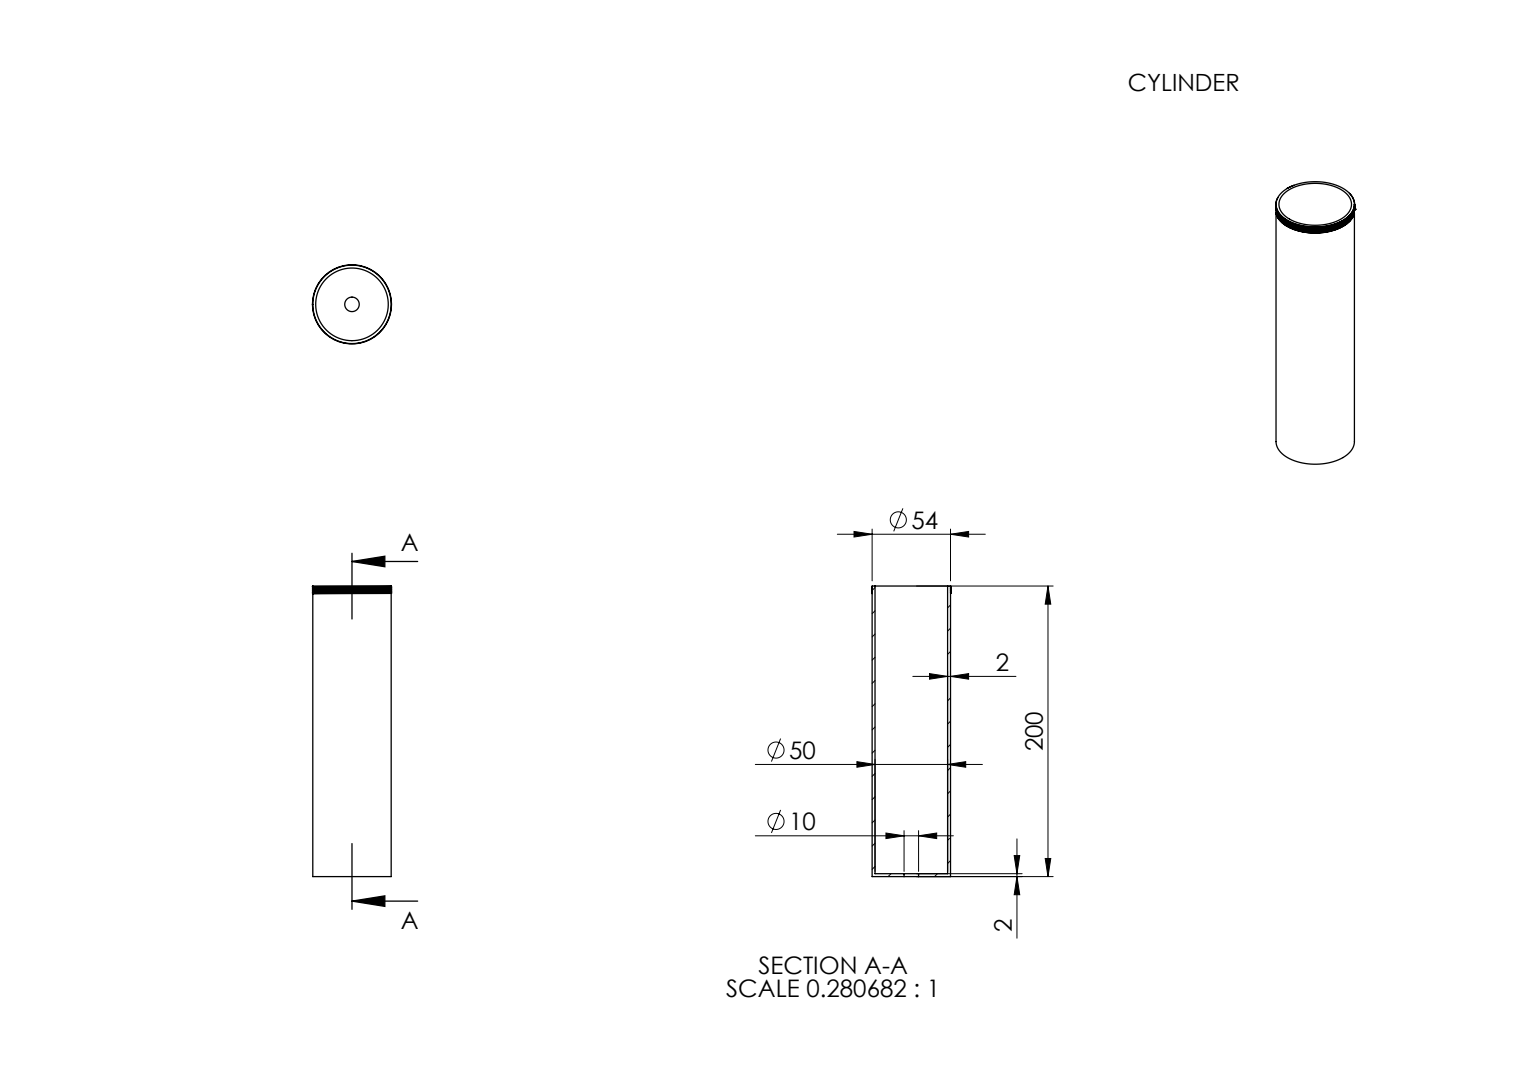
ISO-10303-21;
HEADER;
FILE_DESCRIPTION (('STEP AP214'),
    '1' );
FILE_NAME ('Cylinder.step',
    '2026-10-31T03:36:27',
    ( '' ),
    ( '' ),
    'SwSTEP 2.0',
    'SolidWorks 2026',
    '' );
FILE_SCHEMA (( 'AUTOMOTIVE_DESIGN' ));
ENDSEC;

DATA;
#6=CARTESIAN_POINT ( 'NONE',  ( -3.253724281355068545E-15, 198.6500000012290172, -27.00000000000000355 ) ) ;
#13=CARTESIAN_POINT ( 'NONE',  ( -1.926257025242585782E-15, 198.3968750006145285, -31.45816453501076637 ) ) ;
#14=ORIENTED_EDGE ( 'NONE', *, *, #10865, .F. ) ;
#23=CARTESIAN_POINT ( 'NONE',  ( -13.62178482187500528, 199.2781250006145228, -23.59362340125807123 ) ) ;
#44=CARTESIAN_POINT ( 'NONE',  ( 13.62178482187501416, 195.9593750006145569, 23.59362340125806767 ) ) ;
#51=VECTOR ( 'NONE', #30355, 1000.000000000000000 ) ;
#55=VERTEX_POINT ( 'NONE', #18167 ) ;
#61=CARTESIAN_POINT ( 'NONE',  ( 27.00000000000001066, 196.1375000000000171, 15.58845726811988897 ) ) ;
#84=ORIENTED_EDGE ( 'NONE', *, *, #36303, .T. ) ;
#90=( BOUNDED_CURVE ( )  B_SPLINE_CURVE ( 2, ( #11851, #8830, #29090, #22871, #2761, #17369, #11485, #23054, #34600 ),
 .UNSPECIFIED., .F., .F. ) 
 B_SPLINE_CURVE_WITH_KNOTS ( ( 3, 2, 2, 2, 3 ),
 ( 0.3125000000000000000, 0.3194444444444444198, 0.3333333333333333148, 0.3472222222222222099, 0.3541666666666666852 ),
 .UNSPECIFIED. ) 
 CURVE ( )  GEOMETRIC_REPRESENTATION_ITEM ( )  RATIONAL_B_SPLINE_CURVE ( ( 0.9330127018922194093, 0.9330127018922194093, 1.000000000000000000, 0.8660254037844387076, 1.000000000000000000, 0.8660254037844387076, 1.000000000000000000, 0.9330127018922190762, 0.9330127018922194093 ) ) 
 REPRESENTATION_ITEM ( '' )  );
#93=CARTESIAN_POINT ( 'NONE',  ( 27.24356964375000700, 199.0906250006145228, 15.72908226750537075 ) ) ;
#170=CARTESIAN_POINT ( 'NONE',  ( 5.727106289114498080E-15, 197.0750000012290570, 31.17691453623979214 ) ) ;
#185=CARTESIAN_POINT ( 'NONE',  ( 0.000000000000000000, 2.000000000000000000, 0.000000000000000000 ) ) ;
#199=CARTESIAN_POINT ( 'NONE',  ( 0.000000000000000000, 0.000000000000000000, 0.000000000000000000 ) ) ;
#204=ORIENTED_EDGE ( 'NONE', *, *, #34329, .T. ) ;
#214=CARTESIAN_POINT ( 'NONE',  ( 27.24356964374999635, 199.1656250006145399, -15.72908226750539029 ) ) ;
#226=AXIS2_PLACEMENT_3D ( 'NONE', #11748, #5679, #26519 ) ;
#235=CARTESIAN_POINT ( 'NONE',  ( 13.62178482187501416, 195.0593750006145513, 23.59362340125806767 ) ) ;
#251=CARTESIAN_POINT ( 'NONE',  ( 27.24356964375000345, 198.2843750006145456, -3.336375036156643733E-15 ) ) ;
#256=CARTESIAN_POINT ( 'NONE',  ( -27.00000000000000355, 195.5000000000000000, 0.000000000000000000 ) ) ;
#263=SHAPE_REPRESENTATION_RELATIONSHIP ( 'NONE' , 'NONE' ,  #10836, #22840 ) ;
#296=CARTESIAN_POINT ( 'NONE',  ( 5.727106289114498080E-15, 199.2125000000000057, 31.17691453623979214 ) ) ;
#302=DIRECTION ( 'NONE',  ( -0.000000000000000000, -1.000000000000000000, -0.000000000000000000 ) ) ;
#305=DIRECTION ( 'NONE',  ( 0.000000000000000000, -1.000000000000000000, 0.000000000000000000 ) ) ;
#333=CARTESIAN_POINT ( 'NONE',  ( 26.99999999999999645, 199.8125000000000000, -15.58845726811990495 ) ) ;
#349=ORIENTED_EDGE ( 'NONE', *, *, #34489, .T. ) ;
#357=CARTESIAN_POINT ( 'NONE',  ( 13.49999999999999645, 196.3625000012290513, -23.38268590217984766 ) ) ;
#388=CARTESIAN_POINT ( 'NONE',  ( 27.24356964374999279, 199.2218750006145171, -15.72908226750539207 ) ) ;
#398=CARTESIAN_POINT ( 'NONE',  ( -27.24356964375000345, 198.4531250006145342, 0.000000000000000000 ) ) ;
#420=CARTESIAN_POINT ( 'NONE',  ( 27.24356964375000700, 195.5468750006145342, 15.72908226750537075 ) ) ;
#438=CARTESIAN_POINT ( 'NONE',  ( -27.24356964375000345, 198.0593750006145513, 0.000000000000000000 ) ) ;
#481=CARTESIAN_POINT ( 'NONE',  ( -1.909035429704832693E-15, 199.8875000000000171, -31.17691453623979214 ) ) ;
#539=CARTESIAN_POINT ( 'NONE',  ( 13.50000000000001421, 197.1125000012290513, 23.38268590217984055 ) ) ;
#559=CARTESIAN_POINT ( 'NONE',  ( -27.24356964374999635, 195.8468750006145171, 15.72908226750539384 ) ) ;
#570=CARTESIAN_POINT ( 'NONE',  ( -27.24356964375000345, 198.9218750006145626, -15.72908226750537786 ) ) ;
#580=CARTESIAN_POINT ( 'NONE',  ( -1.926257025242585782E-15, 199.2406250006145285, -31.45816453501075927 ) ) ;
#604=CARTESIAN_POINT ( 'NONE',  ( 27.24356964374999635, 195.6218750006145228, -15.72908226750539029 ) ) ;
#621=CARTESIAN_POINT ( 'NONE',  ( 13.62178482187501416, 197.7593750006145399, 23.59362340125806767 ) ) ;
#665=CARTESIAN_POINT ( 'NONE',  ( -13.50000000000000533, 199.9250000000000114, -23.38268590217984411 ) ) ;
#669=CARTESIAN_POINT ( 'NONE',  ( 0.000000000000000000, 200.0000000000000000, -25.00000000000000000 ) ) ;
#672=CARTESIAN_POINT ( 'NONE',  ( -13.50000000000000533, 198.2375000012290229, -23.38268590217984411 ) ) ;
#725=CARTESIAN_POINT ( 'NONE',  ( 13.49999999999999645, 195.0125000012290570, -23.38268590217984766 ) ) ;
#728=EDGE_CURVE ( 'NONE', #34798, #36105, #17305, .T. ) ;
#748=CARTESIAN_POINT ( 'NONE',  ( 27.24356964375000345, 196.4843750006145626, -3.336375036156643733E-15 ) ) ;
#759=CARTESIAN_POINT ( 'NONE',  ( 0.000000000000000000, 200.0000000000000000, 0.000000000000000000 ) ) ;
#761=CARTESIAN_POINT ( 'NONE',  ( -13.62178482187498396, 196.7843750006145456, 23.59362340125808188 ) ) ;
#774=CARTESIAN_POINT ( 'NONE',  ( 5.778771075727756162E-15, 197.6656250006145399, 31.45816453501075927 ) ) ;
#798=CARTESIAN_POINT ( 'NONE',  ( 13.62178482187501416, 197.7031250006145342, 23.59362340125806767 ) ) ;
#812=CARTESIAN_POINT ( 'NONE',  ( -13.62178482187500528, 197.5343750006145456, -23.59362340125807123 ) ) ;
#813=EDGE_LOOP ( 'NONE', ( #35823, #32630, #11265, #6472 ) ) ;
#817=CARTESIAN_POINT ( 'NONE',  ( -13.49999999999998401, 195.5749999999999886, 23.38268590217985476 ) ) ;
#840=CARTESIAN_POINT ( 'NONE',  ( 27.24356964375000345, 198.6781250006145569, -3.336375036156643733E-15 ) ) ;
#857=CARTESIAN_POINT ( 'NONE',  ( 26.99999999999999645, 199.3625000000000114, -15.58845726811990495 ) ) ;
#872=LINE ( 'NONE', #24196, #29464 ) ;
#896=CARTESIAN_POINT ( 'NONE',  ( 3.306546357697854128E-15, 200.0000000000000000, 27.00000000000000355 ) ) ;
#939=CARTESIAN_POINT ( 'NONE',  ( 5.778771075727756162E-15, 195.0218750006145569, 31.45816453501075927 ) ) ;
#948=CARTESIAN_POINT ( 'NONE',  ( 7.234628195640322446, 198.3325961894323370, 26.99999999999999645 ) ) ;
#950=CARTESIAN_POINT ( 'NONE',  ( -1.926257025242585782E-15, 196.5968750006145456, -31.45816453501076637 ) ) ;
#958=CARTESIAN_POINT ( 'NONE',  ( 3.253724281355069334E-15, 199.5500000012290513, -27.00000000000000000 ) ) ;
#962=CARTESIAN_POINT ( 'NONE',  ( -27.24356964375000345, 196.2031250006145342, 0.000000000000000000 ) ) ;
#985=CARTESIAN_POINT ( 'NONE',  ( 13.62178482187499640, 197.4031250006145228, -23.59362340125807123 ) ) ;
#1023=CARTESIAN_POINT ( 'NONE',  ( 0.000000000000000000, 0.000000000000000000, 0.000000000000000000 ) ) ;
#1027=CARTESIAN_POINT ( 'NONE',  ( 27.24356964374999279, 198.2656250006145058, -15.72908226750539207 ) ) ;
#1039=DIRECTION ( 'NONE',  ( 0.000000000000000000, 0.000000000000000000, -1.000000000000000000 ) ) ;
#1050=CARTESIAN_POINT ( 'NONE',  ( -13.49999999999998401, 198.3875000012290286, 23.38268590217985476 ) ) ;
#1060=EDGE_CURVE ( 'NONE', #37392, #27477, #5776, .T. ) ;
#1101=VERTEX_POINT ( 'NONE', #20197 ) ;
#1124=CARTESIAN_POINT ( 'NONE',  ( -27.00000000000000355, 199.0625000000000000, -15.58845726811989429 ) ) ;
#1128=CARTESIAN_POINT ( 'NONE',  ( -13.62178482187500528, 195.2843750006145456, -23.59362340125807123 ) ) ;
#1135=CARTESIAN_POINT ( 'NONE',  ( 7.234628195640312676, 199.5299038117966859, -27.00000000000000711 ) ) ;
#1136=CARTESIAN_POINT ( 'NONE',  ( 7.234628195640322446, 198.7825961894323257, 26.99999999999999645 ) ) ;
#1138=CARTESIAN_POINT ( 'NONE',  ( -13.62178482187498396, 196.3343750006145285, 23.59362340125808188 ) ) ;
#1139=ORIENTED_EDGE ( 'NONE', *, *, #3630, .F. ) ;
#1150=EDGE_LOOP ( 'NONE', ( #1703, #18410, #14, #35728 ) ) ;
#1151=CARTESIAN_POINT ( 'NONE',  ( -27.24356964375000345, 195.7531250006145456, 0.000000000000000000 ) ) ;
#1174=CARTESIAN_POINT ( 'NONE',  ( -13.62178482187500528, 199.7281250006145399, -23.59362340125807123 ) ) ;
#1177=DIRECTION ( 'NONE',  ( -0.000000000000000000, -1.000000000000000000, -0.000000000000000000 ) ) ;
#1188=ORIENTED_EDGE ( 'NONE', *, *, #28113, .F. ) ;
#1209=CARTESIAN_POINT ( 'NONE',  ( -7.234628195640316228, 197.3200961906614168, -27.00000000000000000 ) ) ;
#1212=CARTESIAN_POINT ( 'NONE',  ( -27.24356964375000345, 197.9656250006145797, -15.72908226750537786 ) ) ;
#1228=CARTESIAN_POINT ( 'NONE',  ( 13.50000000000001421, 198.8000000000000114, 23.38268590217984055 ) ) ;
#1242=ADVANCED_FACE ( 'NONE', ( #35518 ), #20758, .F. ) ;
#1258=CARTESIAN_POINT ( 'NONE',  ( -1.045839947578415010E-13, 196.1750000012290229, 27.00000000000000355 ) ) ;
#1318=VERTEX_POINT ( 'NONE', #35323 ) ;
#1325=CARTESIAN_POINT ( 'NONE',  ( 27.00000000000000355, 199.4375000012290400, -3.306546357697854128E-15 ) ) ;
#1329=CARTESIAN_POINT ( 'NONE',  ( 27.24356964375000700, 195.9968750006145513, 15.72908226750537075 ) ) ;
#1341=CARTESIAN_POINT ( 'NONE',  ( -27.24356964375000345, 196.6531250006145513, 0.000000000000000000 ) ) ;
#1352=FACE_OUTER_BOUND ( 'NONE', #34745, .T. ) ;
#1367=CARTESIAN_POINT ( 'NONE',  ( -27.24356964374999990, 198.8656250006145569, -15.72908226750537786 ) ) ;
#1371=EDGE_CURVE ( 'NONE', #27477, #5428, #18984, .T. ) ;
#1396=CARTESIAN_POINT ( 'NONE',  ( -27.00000000000000355, 198.1625000000000227, -15.58845726811989429 ) ) ;
#1403=CARTESIAN_POINT ( 'NONE',  ( -1.926257025242585782E-15, 198.3406250006145228, -31.45816453501076637 ) ) ;
#1418=CARTESIAN_POINT ( 'NONE',  ( -26.99999999999998934, 196.4375000000000284, 15.58845726811991561 ) ) ;
#1476=ORIENTED_EDGE ( 'NONE', *, *, #2642, .F. ) ;
#1484=CARTESIAN_POINT ( 'NONE',  ( -1.909035429704832693E-15, 195.0500000012290229, -31.17691453623979214 ) ) ;
#1492=CARTESIAN_POINT ( 'NONE',  ( 13.50000000000001421, 196.1000000000000227, 23.38268590217984055 ) ) ;
#1497=DIRECTION ( 'NONE',  ( -0.000000000000000000, -1.000000000000000000, -0.000000000000000000 ) ) ;
#1513=CARTESIAN_POINT ( 'NONE',  ( 27.24356964374999279, 196.5218750006145569, -15.72908226750539207 ) ) ;
#1520=( BOUNDED_CURVE ( )  B_SPLINE_CURVE ( 2, ( #4940, #16154, #15967, #30924, #13483, #25039, #33392, #36780, #7432 ),
 .UNSPECIFIED., .F., .F. ) 
 B_SPLINE_CURVE_WITH_KNOTS ( ( 3, 2, 2, 2, 3 ),
 ( 0.1041666666666666713, 0.1111111111111111049, 0.1250000000000000000, 0.1388888888888888951, 0.1458333333333333426 ),
 .UNSPECIFIED. ) 
 CURVE ( )  GEOMETRIC_REPRESENTATION_ITEM ( )  RATIONAL_B_SPLINE_CURVE ( ( 0.9330127018922194093, 0.9330127018922194093, 1.000000000000000000, 0.8660254037844387076, 1.000000000000000000, 0.8660254037844387076, 1.000000000000000000, 0.9330127018922194093, 0.9330127018922194093 ) ) 
 REPRESENTATION_ITEM ( '' )  );
#1525=CARTESIAN_POINT ( 'NONE',  ( -27.24356964375000345, 197.1031250006145399, 0.000000000000000000 ) ) ;
#1540=DIRECTION ( 'NONE',  ( 0.000000000000000000, -1.000000000000000000, 0.000000000000000000 ) ) ;
#1547=ORIENTED_EDGE ( 'NONE', *, *, #13873, .F. ) ;
#1548=LINE ( 'NONE', #19197, #28798 ) ;
#1552=CARTESIAN_POINT ( 'NONE',  ( -1.926257025242585782E-15, 199.6906250006145456, -31.45816453501075927 ) ) ;
#1565=AXIS2_PLACEMENT_3D ( 'NONE', #36851, #23023, #17153 ) ;
#1580=CARTESIAN_POINT ( 'NONE',  ( 13.50000000000001421, 195.7625000012290570, 23.38268590217984055 ) ) ;
#1593=CARTESIAN_POINT ( 'NONE',  ( -1.926257025242585782E-15, 196.5406250006145399, -31.45816453501076637 ) ) ;
#1595=DIRECTION ( 'NONE',  ( 0.000000000000000000, 0.000000000000000000, -1.000000000000000000 ) ) ;
#1598=CARTESIAN_POINT ( 'NONE',  ( 27.00000000000001421, 196.2500000012290116, 15.58845726811988897 ) ) ;
#1609=CARTESIAN_POINT ( 'NONE',  ( 26.99999999999999645, 198.4625000000000341, -15.58845726811990495 ) ) ;
#1617=CARTESIAN_POINT ( 'NONE',  ( -27.00000000000000355, 196.3625000000000114, -15.58845726811989429 ) ) ;
#1641=DIRECTION ( 'NONE',  ( -0.000000000000000000, -1.000000000000000000, -0.000000000000000000 ) ) ;
#1655=CARTESIAN_POINT ( 'NONE',  ( 6.123233995736766282E-16, 0.000000000000000000, 5.000000000000000000 ) ) ;
#1665=EDGE_LOOP ( 'NONE', ( #22970, #4177, #13653, #15801, #24714, #31155, #33788, #28685 ) ) ;
#1684=CARTESIAN_POINT ( 'NONE',  ( -13.49999999999998401, 195.6875000012290400, 23.38268590217985476 ) ) ;
#1686=DIRECTION ( 'NONE',  ( -0.000000000000000000, -1.000000000000000000, -0.000000000000000000 ) ) ;
#1701=CARTESIAN_POINT ( 'NONE',  ( 5.778771075727756162E-15, 195.9218750006145342, 31.45816453501076637 ) ) ;
#1703=ORIENTED_EDGE ( 'NONE', *, *, #14020, .T. ) ;
#1714=CARTESIAN_POINT ( 'NONE',  ( -27.24356964375001056, 194.8294844423495533, -9.915847621322177119 ) ) ;
#1731=CARTESIAN_POINT ( 'NONE',  ( 13.49999999999999645, 198.0500000000000114, -23.38268590217984766 ) ) ;
#1735=ORIENTED_EDGE ( 'NONE', *, *, #15718, .F. ) ;
#1740=CARTESIAN_POINT ( 'NONE',  ( -13.62178482187500528, 197.0281250006145228, -23.59362340125807123 ) ) ;
#1744=DIRECTION ( 'NONE',  ( 0.000000000000000000, 0.000000000000000000, -1.000000000000000000 ) ) ;
#1761=( BOUNDED_CURVE ( )  B_SPLINE_CURVE ( 2, ( #33202, #15774, #36034, #10078, #28067, #7429, #33389, #27880, #10632 ),
 .UNSPECIFIED., .F., .F. ) 
 B_SPLINE_CURVE_WITH_KNOTS ( ( 3, 2, 2, 2, 3 ),
 ( 0.7708333333333333703, 0.7777777777777777901, 0.7916666666666666297, 0.8055555555555555802, 0.8125000000000000000 ),
 .UNSPECIFIED. ) 
 CURVE ( )  GEOMETRIC_REPRESENTATION_ITEM ( )  RATIONAL_B_SPLINE_CURVE ( ( 0.9330127018922192983, 0.9330127018922198534, 1.000000000000000000, 0.8660254037844387076, 1.000000000000000000, 0.8660254037844387076, 1.000000000000000000, 0.9330127018922194093, 0.9330127018922194093 ) ) 
 REPRESENTATION_ITEM ( '' )  );
#1780=CARTESIAN_POINT ( 'NONE',  ( -13.62178482187498396, 195.3781250006145171, 23.59362340125808188 ) ) ;
#1781=CARTESIAN_POINT ( 'NONE',  ( -27.24356964375000345, 197.1593750006145456, 0.000000000000000000 ) ) ;
#1791=ADVANCED_FACE ( 'NONE', ( #17077 ), #6254, .F. ) ;
#1796=CARTESIAN_POINT ( 'NONE',  ( 13.50000000000001421, 198.3499999999999943, 23.38268590217984055 ) ) ;
#1837=CARTESIAN_POINT ( 'NONE',  ( 27.00000000000000355, 197.6375000012290286, -3.306546357697854128E-15 ) ) ;
#1851=VERTEX_POINT ( 'NONE', #11381 ) ;
#1901=CARTESIAN_POINT ( 'NONE',  ( -13.49999999999998401, 198.3875000012290286, 23.38268590217985476 ) ) ;
#1914=UNCERTAINTY_MEASURE_WITH_UNIT (LENGTH_MEASURE( 1.000000000000000082E-05 ), #7486, 'distance_accuracy_value', 'NONE');
#1915=DIRECTION ( 'NONE',  ( 0.000000000000000000, 1.000000000000000000, 0.000000000000000000 ) ) ;
#1923=CARTESIAN_POINT ( 'NONE',  ( 27.24356964375000700, 195.4906250006145001, 15.72908226750537075 ) ) ;
#1963=CARTESIAN_POINT ( 'NONE',  ( 27.24356964374999635, 197.8718750006145513, -15.72908226750539029 ) ) ;
#1979=CARTESIAN_POINT ( 'NONE',  ( 13.49999999999999645, 197.5999999999999943, -23.38268590217984766 ) ) ;
#2005=EDGE_LOOP ( 'NONE', ( #16646, #26117 ) ) ;
#2032=DIRECTION ( 'NONE',  ( 0.000000000000000000, 0.000000000000000000, -1.000000000000000000 ) ) ;
#2044=CARTESIAN_POINT ( 'NONE',  ( 1.255007937094097924E-14, 199.4375000000000284, -27.00000000000000000 ) ) ;
#2065=CARTESIAN_POINT ( 'NONE',  ( -26.99999999999999645, 197.3375000000000057, 15.58845726811991561 ) ) ;
#2078=CARTESIAN_POINT ( 'NONE',  ( 5.778771075727756162E-15, 195.4718750006145171, 31.45816453501076637 ) ) ;
#2081=CARTESIAN_POINT ( 'NONE',  ( 26.99999999999999645, 196.7750000012290172, -15.58845726811990495 ) ) ;
#2090=EDGE_LOOP ( 'NONE', ( #4509, #18606, #4185, #1735 ) ) ;
#2091=CARTESIAN_POINT ( 'NONE',  ( 26.99999999999999645, 199.0250000012290457, -15.58845726811990495 ) ) ;
#2111=CARTESIAN_POINT ( 'NONE',  ( 13.62178482187501416, 195.0031250006145456, 23.59362340125806767 ) ) ;
#2137=CARTESIAN_POINT ( 'NONE',  ( -1.045839947578415010E-13, 195.7250000012290343, 27.00000000000000355 ) ) ;
#2145=CARTESIAN_POINT ( 'NONE',  ( -1.045839947578415010E-13, 194.8250000012290570, 27.00000000000000355 ) ) ;
#2148=CARTESIAN_POINT ( 'NONE',  ( -1.926257025242585782E-15, 195.6406250006145342, -31.45816453501076637 ) ) ;
#2149=CARTESIAN_POINT ( 'NONE',  ( 13.62178482187499640, 197.4593750006145285, -23.59362340125807123 ) ) ;
#2152=CARTESIAN_POINT ( 'NONE',  ( 1.120210788295102201E-13, 196.4000000012290741, -27.00000000000000711 ) ) ;
#2164=CARTESIAN_POINT ( 'NONE',  ( 26.99999999999999645, 196.2125000000000057, -15.58845726811990495 ) ) ;
#2205=CARTESIAN_POINT ( 'NONE',  ( 7.234628195640295800, 197.5450961906613827, 27.00000000000001066 ) ) ;
#2239=FACE_OUTER_BOUND ( 'NONE', #20647, .T. ) ;
#2257=CARTESIAN_POINT ( 'NONE',  ( 0.000000000000000000, 200.0000000000000000, 0.000000000000000000 ) ) ;
#2265=B_SPLINE_CURVE_WITH_KNOTS ( 'NONE', 3,
 ( #22801, #8950, #17115, #34351 ),
 .UNSPECIFIED., .F., .F.,
 ( 4, 4 ),
 ( 0.000000000000000000, 1.000000000000000000 ),
 .UNSPECIFIED. ) ;
#2270=DIRECTION ( 'NONE',  ( -0.000000000000000000, -1.000000000000000000, -0.000000000000000000 ) ) ;
#2274=CARTESIAN_POINT ( 'NONE',  ( -13.50000000000000533, 199.1375000012290286, -23.38268590217984411 ) ) ;
#2294=ORIENTED_EDGE ( 'NONE', *, *, #16417, .T. ) ;
#2298=CARTESIAN_POINT ( 'NONE',  ( 27.24356964375000700, 195.9406250006145456, 15.72908226750537075 ) ) ;
#2314=EDGE_CURVE ( 'NONE', #21803, #18034, #2265, .T. ) ;
#2327=ORIENTED_EDGE ( 'NONE', *, *, #19803, .F. ) ;
#2337=CARTESIAN_POINT ( 'NONE',  ( 13.50000000000001421, 194.8625000012290513, 23.38268590217984055 ) ) ;
#2340=CARTESIAN_POINT ( 'NONE',  ( -27.24356964375000700, 194.8294844423495817, -9.915847621322177119 ) ) ;
#2341=CARTESIAN_POINT ( 'NONE',  ( 27.24356964375000700, 199.1468750006145285, 15.72908226750537075 ) ) ;
#2355=DIRECTION ( 'NONE',  ( 0.000000000000000000, 0.000000000000000000, -1.000000000000000000 ) ) ;
#2356=CARTESIAN_POINT ( 'NONE',  ( -1.909035429704832693E-15, 196.2875000000000227, -31.17691453623979214 ) ) ;
#2455=DIRECTION ( 'NONE',  ( 0.000000000000000000, 0.000000000000000000, -1.000000000000000000 ) ) ;
#2458=CARTESIAN_POINT ( 'NONE',  ( -20.86978604919638869, 194.8026013911397740, -17.51182792271053046 ) ) ;
#2464=DIRECTION ( 'NONE',  ( -0.000000000000000000, -1.000000000000000000, -0.000000000000000000 ) ) ;
#2482=CARTESIAN_POINT ( 'NONE',  ( 13.62178482187499640, 195.1531250006145513, -23.59362340125807123 ) ) ;
#2489=ORIENTED_EDGE ( 'NONE', *, *, #31608, .T. ) ;
#2526=CARTESIAN_POINT ( 'NONE',  ( -27.24356964374999990, 197.5718750006145399, -15.72908226750537786 ) ) ;
#2529=CARTESIAN_POINT ( 'NONE',  ( 26.99999999999999645, 195.7625000000000171, -15.58845726811990495 ) ) ;
#2537=CARTESIAN_POINT ( 'NONE',  ( 7.234628195640295800, 197.0950961906613941, 27.00000000000001066 ) ) ;
#2543=CARTESIAN_POINT ( 'NONE',  ( -26.99999999999998934, 195.9875000000000114, 15.58845726811991561 ) ) ;
#2577=CARTESIAN_POINT ( 'NONE',  ( 0.000000000000000000, 0.000000000000000000, 0.000000000000000000 ) ) ;
#2631=VERTEX_POINT ( 'NONE', #27747 ) ;
#2639=CARTESIAN_POINT ( 'NONE',  ( -13.50000000000000533, 197.3375000012290457, -23.38268590217984411 ) ) ;
#2642=EDGE_CURVE ( 'NONE', #34685, #32085, #8558, .T. ) ;
#2665=CARTESIAN_POINT ( 'NONE',  ( -20.86978606573367045, 194.8588513912095266, -17.51182790300216752 ) ) ;
#2668=DIRECTION ( 'NONE',  ( 0.000000000000000000, 0.000000000000000000, -1.000000000000000000 ) ) ;
#2672=CARTESIAN_POINT ( 'NONE',  ( 13.62178482187501416, 198.6593750006145456, 23.59362340125806767 ) ) ;
#2686=DIRECTION ( 'NONE',  ( -0.000000000000000000, -1.000000000000000000, -0.000000000000000000 ) ) ;
#2701=CARTESIAN_POINT ( 'NONE',  ( -13.50000000000000533, 198.6875000012290400, -23.38268590217984411 ) ) ;
#2702=CARTESIAN_POINT ( 'NONE',  ( 13.62178482187499640, 196.1093750006145342, -23.59362340125807123 ) ) ;
#2704=CARTESIAN_POINT ( 'NONE',  ( -27.00000000000000355, 198.6125000000000114, -15.58845726811989429 ) ) ;
#2713=CARTESIAN_POINT ( 'NONE',  ( -26.99999999999999645, 195.9875000000000114, 15.58845726811991561 ) ) ;
#2719=VECTOR ( 'NONE', #15417, 1000.000000000000000 ) ;
#2722=CARTESIAN_POINT ( 'NONE',  ( 13.50000000000001421, 196.1000000000000227, 23.38268590217984055 ) ) ;
#2732=EDGE_CURVE ( 'NONE', #10880, #4926, #27922, .T. ) ;
#2761=CARTESIAN_POINT ( 'NONE',  ( -27.00000000000000355, 197.8625000012290513, 0.000000000000000000 ) ) ;
#2775=VERTEX_POINT ( 'NONE', #5174 ) ;
#2781=CARTESIAN_POINT ( 'NONE',  ( 0.000000000000000000, 2.000000000000000000, -5.000000000000000000 ) ) ;
#2804=AXIS2_PLACEMENT_3D ( 'NONE', #21586, #33689, #2032 ) ;
#2808=ORIENTED_EDGE ( 'NONE', *, *, #7091, .T. ) ;
#2826=CARTESIAN_POINT ( 'NONE',  ( 27.00000000000001066, 197.1500000012290172, 15.58845726811988897 ) ) ;
#2866=CARTESIAN_POINT ( 'NONE',  ( -27.24356964374999635, 198.4906250006145569, 15.72908226750539384 ) ) ;
#2886=CARTESIAN_POINT ( 'NONE',  ( 13.50000000000001421, 195.2000000000000171, 23.38268590217984055 ) ) ;
#2888=CARTESIAN_POINT ( 'NONE',  ( 27.24356964375000700, 196.4468750006145115, 15.72908226750537075 ) ) ;
#2908=CARTESIAN_POINT ( 'NONE',  ( -27.00000000000000355, 195.5000000000000000, 0.000000000000000000 ) ) ;
#2916=EDGE_CURVE ( 'NONE', #24650, #4030, #22848, .T. ) ;
#2957=CARTESIAN_POINT ( 'NONE',  ( -13.50000000000000533, 196.4375000012290400, -23.38268590217984411 ) ) ;
#2974=( BOUNDED_CURVE ( )  B_SPLINE_CURVE ( 2, ( #13003, #16223, #10152, #12806, #15662, #10338, #36478, #25112, #10519 ),
 .UNSPECIFIED., .F., .F. ) 
 B_SPLINE_CURVE_WITH_KNOTS ( ( 3, 2, 2, 2, 3 ),
 ( 0.06250000000000000000, 0.06944444444444444753, 0.08333333333333332871, 0.09722222222222222376, 0.1041666666666666713 ),
 .UNSPECIFIED. ) 
 CURVE ( )  GEOMETRIC_REPRESENTATION_ITEM ( )  RATIONAL_B_SPLINE_CURVE ( ( 0.9330127018922194093, 0.9330127018922194093, 1.000000000000000000, 0.8660254037844387076, 1.000000000000000000, 0.8660254037844387076, 1.000000000000000000, 0.9330127018922192983, 0.9330127018922194093 ) ) 
 REPRESENTATION_ITEM ( '' )  );
#3015=CARTESIAN_POINT ( 'NONE',  ( 27.00000000000001066, 197.6000000012290627, 15.58845726811988897 ) ) ;
#3039=CARTESIAN_POINT ( 'NONE',  ( -27.24356964375000345, 194.8531250006145115, 0.000000000000000000 ) ) ;
#3056=CARTESIAN_POINT ( 'NONE',  ( 13.62178482187499640, 198.3031250006145285, -23.59362340125807123 ) ) ;
#3077=CARTESIAN_POINT ( 'NONE',  ( 13.49999999999999645, 195.3500000000000227, -23.38268590217984766 ) ) ;
#3078=CARTESIAN_POINT ( 'NONE',  ( -27.24356964375000345, 195.3593750006145342, 0.000000000000000000 ) ) ;
#3089=CARTESIAN_POINT ( 'NONE',  ( 13.50000000000001421, 197.1125000012290513, 23.38268590217984055 ) ) ;
#3096=CARTESIAN_POINT ( 'NONE',  ( -13.62178482187498396, 198.1343750006145399, 23.59362340125808188 ) ) ;
#3097=ORIENTED_EDGE ( 'NONE', *, *, #28113, .T. ) ;
#3125=CARTESIAN_POINT ( 'NONE',  ( -27.24356964375000345, 198.8656250006145285, -15.72908226750537786 ) ) ;
#3136=VERTEX_POINT ( 'NONE', #22541 ) ;
#3144=CARTESIAN_POINT ( 'NONE',  ( -7.234628195640263826, 196.4200961906613543, -27.00000000000003553 ) ) ;
#3199=CARTESIAN_POINT ( 'NONE',  ( -27.00000000000000355, 196.0625000012290400, 0.000000000000000000 ) ) ;
#3206=MECHANICAL_DESIGN_GEOMETRIC_PRESENTATION_REPRESENTATION('',(#5694),#13523);
#3211=EDGE_CURVE ( 'NONE', #24650, #1318, #22173, .T. ) ;
#3221=CARTESIAN_POINT ( 'NONE',  ( 13.62178482187501416, 195.0593750006145513, 23.59362340125806767 ) ) ;
#3233=CARTESIAN_POINT ( 'NONE',  ( -1.926257025242585782E-15, 199.2968750006145342, -31.45816453501076637 ) ) ;
#3243=ORIENTED_EDGE ( 'NONE', *, *, #2916, .F. ) ;
#3245=CARTESIAN_POINT ( 'NONE',  ( -27.24356964374999990, 199.7656250006145342, -15.72908226750537786 ) ) ;
#3257=( GEOMETRIC_REPRESENTATION_CONTEXT ( 3 ) GLOBAL_UNCERTAINTY_ASSIGNED_CONTEXT ( ( #1914 ) ) GLOBAL_UNIT_ASSIGNED_CONTEXT ( ( #7486, #36656, #30615 ) ) REPRESENTATION_CONTEXT ( 'NONE', 'WORKASPACE' ) );
#3264=ORIENTED_EDGE ( 'NONE', *, *, #2916, .T. ) ;
#3268=CARTESIAN_POINT ( 'NONE',  ( 27.24356964375000345, 195.5843750006145285, -3.336375036156643733E-15 ) ) ;
#3284=CARTESIAN_POINT ( 'NONE',  ( 5.778771075727756162E-15, 198.1718750006145342, 31.45816453501075927 ) ) ;
#3311=CARTESIAN_POINT ( 'NONE',  ( -13.62178482187500528, 198.8281250006145342, -23.59362340125807123 ) ) ;
#3316=DIRECTION ( 'NONE',  ( -0.000000000000000000, -1.000000000000000000, -0.000000000000000000 ) ) ;
#3329=CARTESIAN_POINT ( 'NONE',  ( 5.727106289114498080E-15, 199.6625000000000227, 31.17691453623979214 ) ) ;
#3335=CARTESIAN_POINT ( 'NONE',  ( 1.069080835302379631E-14, 198.4250000012290229, 27.00000000000000000 ) ) ;
#3376=CARTESIAN_POINT ( 'NONE',  ( 13.50000000000001421, 196.5500000000000114, 23.38268590217984055 ) ) ;
#3386=ADVANCED_FACE ( 'NONE', ( #28394 ), #5091, .T. ) ;
#3392=CARTESIAN_POINT ( 'NONE',  ( 26.99999999999999645, 195.4250000012290229, -15.58845726811990495 ) ) ;
#3410=CARTESIAN_POINT ( 'NONE',  ( 27.24356964375000700, 196.4468750006145115, 15.72908226750537075 ) ) ;
#3422=CARTESIAN_POINT ( 'NONE',  ( -27.24356964374999279, 198.9968750006145513, 15.72908226750539384 ) ) ;
#3432=CARTESIAN_POINT ( 'NONE',  ( -27.24356964375000345, 198.0031250006145456, 0.000000000000000000 ) ) ;
#3449=ORIENTED_EDGE ( 'NONE', *, *, #26598, .T. ) ;
#3454=CARTESIAN_POINT ( 'NONE',  ( -7.234628195640316228, 198.6700961906613543, -27.00000000000000000 ) ) ;
#3456=CARTESIAN_POINT ( 'NONE',  ( 27.24356964375000700, 195.0968750006145456, 15.72908226750537075 ) ) ;
#3474=CARTESIAN_POINT ( 'NONE',  ( -27.24356964374999635, 197.6468750006145285, 15.72908226750539384 ) ) ;
#3476=ORIENTED_EDGE ( 'NONE', *, *, #22471, .T. ) ;
#3495=LINE ( 'NONE', #20761, #21688 ) ;
#3500=CARTESIAN_POINT ( 'NONE',  ( -27.24356964375000345, 199.3531250006145399, 0.000000000000000000 ) ) ;
#3510=ORIENTED_EDGE ( 'NONE', *, *, #36113, .F. ) ;
#3575=ORIENTED_EDGE ( 'NONE', *, *, #31144, .F. ) ;
#3602=CARTESIAN_POINT ( 'NONE',  ( 27.24356964375000345, 195.1343750006145399, -3.336375036156643733E-15 ) ) ;
#3612=CYLINDRICAL_SURFACE ( 'NONE', #31490, 27.00000000000000355 ) ;
#3614=CARTESIAN_POINT ( 'NONE',  ( -27.24356964375000345, 197.5718750006145115, -15.72908226750537786 ) ) ;
#3624=CARTESIAN_POINT ( 'NONE',  ( -13.62178482187500528, 197.9281250006145569, -23.59362340125807123 ) ) ;
#3630=EDGE_CURVE ( 'NONE', #34798, #17216, #32174, .T. ) ;
#3632=CARTESIAN_POINT ( 'NONE',  ( 13.50000000000001421, 197.0000000000000000, 23.38268590217984055 ) ) ;
#3648=CARTESIAN_POINT ( 'NONE',  ( -27.24356964375000345, 198.0031250006145456, 0.000000000000000000 ) ) ;
#3653=DIRECTION ( 'NONE',  ( -0.000000000000000000, -1.000000000000000000, -0.000000000000000000 ) ) ;
#3661=CARTESIAN_POINT ( 'NONE',  ( -1.926257025242585782E-15, 197.0468750006145626, -31.45816453501075927 ) ) ;
#3691=LINE ( 'NONE', #12410, #22908 ) ;
#3782=CARTESIAN_POINT ( 'NONE',  ( 27.24356964375000700, 196.8968750006145285, 15.72908226750537075 ) ) ;
#3784=ORIENTED_EDGE ( 'NONE', *, *, #36113, .T. ) ;
#3793=CARTESIAN_POINT ( 'NONE',  ( -13.62178482187500528, 197.0843750006145285, -23.59362340125807123 ) ) ;
#3794=ORIENTED_EDGE ( 'NONE', *, *, #27314, .F. ) ;
#3806=CARTESIAN_POINT ( 'NONE',  ( -1.926257025242585782E-15, 196.9906250006145569, -31.45816453501075927 ) ) ;
#3833=CARTESIAN_POINT ( 'NONE',  ( -13.62178482187500528, 197.4781250006145399, -23.59362340125807123 ) ) ;
#3834=CARTESIAN_POINT ( 'NONE',  ( 27.00000000000000355, 198.0875000012290457, -3.306546357697854128E-15 ) ) ;
#3863=AXIS2_PLACEMENT_3D ( 'NONE', #4306, #27809, #31209 ) ;
#3875=CARTESIAN_POINT ( 'NONE',  ( 27.24356964375000700, 197.2906250006145399, 15.72908226750537075 ) ) ;
#3887=CARTESIAN_POINT ( 'NONE',  ( 0.000000000000000000, 200.0000000000000000, 0.000000000000000000 ) ) ;
#3894=CARTESIAN_POINT ( 'NONE',  ( 13.50000000000001421, 199.2500000000000000, 23.38268590217984055 ) ) ;
#3897=ORIENTED_EDGE ( 'NONE', *, *, #19583, .F. ) ;
#3900=FACE_OUTER_BOUND ( 'NONE', #18753, .T. ) ;
#3941=ADVANCED_FACE ( 'NONE', ( #18546 ), #26670, .F. ) ;
#3953=CARTESIAN_POINT ( 'NONE',  ( -27.00000000000000355, 195.1625000012290343, 0.000000000000000000 ) ) ;
#3970=CARTESIAN_POINT ( 'NONE',  ( 26.99999999999999645, 199.0250000012290172, -15.58845726811990495 ) ) ;
#3973=CARTESIAN_POINT ( 'NONE',  ( -27.24356964374999635, 196.7468750006145797, 15.72908226750539384 ) ) ;
#3982=CARTESIAN_POINT ( 'NONE',  ( 27.00000000000000355, 198.4250000000000114, -3.306546357697854128E-15 ) ) ;
#3984=CARTESIAN_POINT ( 'NONE',  ( -13.62178482187498396, 198.1343750006145399, 23.59362340125808188 ) ) ;
#3993=ORIENTED_EDGE ( 'NONE', *, *, #36975, .T. ) ;
#3996=CARTESIAN_POINT ( 'NONE',  ( 27.24356964374999635, 196.0156250006145626, -15.72908226750539029 ) ) ;
#4023=CARTESIAN_POINT ( 'NONE',  ( -13.62178482187498396, 198.9781250006145399, 23.59362340125808188 ) ) ;
#4024=CYLINDRICAL_SURFACE ( 'NONE', #12318, 27.00000000000000355 ) ;
#4030=VERTEX_POINT ( 'NONE', #24216 ) ;
#4056=CARTESIAN_POINT ( 'NONE',  ( -7.234628195640289583, 198.1075961894323143, -27.00000000000001421 ) ) ;
#4064=CARTESIAN_POINT ( 'NONE',  ( -27.24356964375000345, 198.0031250006145456, 0.000000000000000000 ) ) ;
#4066=LINE ( 'NONE', #10130, #20503 ) ;
#4090=CARTESIAN_POINT ( 'NONE',  ( -7.234628195640302017, 198.4049038117967143, 27.00000000000000711 ) ) ;
#4118=DIRECTION ( 'NONE',  ( 0.000000000000000000, 0.000000000000000000, -1.000000000000000000 ) ) ;
#4145=CARTESIAN_POINT ( 'NONE',  ( 5.727106289114498080E-15, 195.2750000012290172, 31.17691453623979214 ) ) ;
#4176=CARTESIAN_POINT ( 'NONE',  ( 27.24356964374999279, 196.0718750006145399, -15.72908226750539207 ) ) ;
#4177=ORIENTED_EDGE ( 'NONE', *, *, #27306, .T. ) ;
#4183=( BOUNDED_CURVE ( )  B_SPLINE_CURVE ( 2, ( #2152, #5183, #10876, #27568, #11062, #1598, #34184, #22265, #33439 ),
 .UNSPECIFIED., .F., .F. ) 
 B_SPLINE_CURVE_WITH_KNOTS ( ( 3, 2, 2, 2, 3 ),
 ( 0.6041666666666667407, 0.6111111111111111605, 0.6250000000000000000, 0.6388888888888888395, 0.6458333333333333703 ),
 .UNSPECIFIED. ) 
 CURVE ( )  GEOMETRIC_REPRESENTATION_ITEM ( )  RATIONAL_B_SPLINE_CURVE ( ( 0.9330127018922192983, 0.9330127018922198534, 1.000000000000000000, 0.8660254037844387076, 1.000000000000000000, 0.8660254037844387076, 1.000000000000000000, 0.9330127018922187432, 0.9330127018922192983 ) ) 
 REPRESENTATION_ITEM ( '' )  );
#4185=ORIENTED_EDGE ( 'NONE', *, *, #35475, .F. ) ;
#4188=CARTESIAN_POINT ( 'NONE',  ( 27.24356964375000345, 195.9781250006145399, -3.336375036156643733E-15 ) ) ;
#4210=CARTESIAN_POINT ( 'NONE',  ( 27.24356964374999635, 198.7156250006145513, -15.72908226750539029 ) ) ;
#4211=CARTESIAN_POINT ( 'NONE',  ( -27.00000000000000355, 200.0000000000000000, 0.000000000000000000 ) ) ;
#4249=CARTESIAN_POINT ( 'NONE',  ( -27.24356964375000345, 197.1031250006145399, 0.000000000000000000 ) ) ;
#4253=CARTESIAN_POINT ( 'NONE',  ( -1.045839947578415010E-13, 195.1625000000000512, 27.00000000000000355 ) ) ;
#4265=CARTESIAN_POINT ( 'NONE',  ( 27.00000000000000355, 197.5250000000000057, -3.306546357697854128E-15 ) ) ;
#4288=DIRECTION ( 'NONE',  ( 0.000000000000000000, -1.000000000000000000, 0.000000000000000000 ) ) ;
#4306=CARTESIAN_POINT ( 'NONE',  ( 0.000000000000000000, 200.0000000000000000, 0.000000000000000000 ) ) ;
#4320=AXIS2_PLACEMENT_3D ( 'NONE', #185, #22254, #37331 ) ;
#4328=CARTESIAN_POINT ( 'NONE',  ( 27.00000000000001066, 194.9000000012290457, 15.58845726811988897 ) ) ;
#4349=EDGE_LOOP ( 'NONE', ( #10680, #4641, #36463, #13800 ) ) ;
#4358=CARTESIAN_POINT ( 'NONE',  ( 27.24356964375000700, 197.3468750006145740, 15.72908226750537075 ) ) ;
#4371=ORIENTED_EDGE ( 'NONE', *, *, #15199, .F. ) ;
#4372=CARTESIAN_POINT ( 'NONE',  ( -13.62178482187498396, 197.1781250006145569, 23.59362340125808188 ) ) ;
#4383=VERTEX_POINT ( 'NONE', #37250 ) ;
#4395=CARTESIAN_POINT ( 'NONE',  ( 5.778771075727756162E-15, 197.6656250006145399, 31.45816453501075927 ) ) ;
#4416=( BOUNDED_CURVE ( )  B_SPLINE_CURVE ( 2, ( #6515, #14670, #817, #26220, #256, #11821, #23390, #20555, #37156 ),
 .UNSPECIFIED., .F., .F. ) 
 B_SPLINE_CURVE_WITH_KNOTS ( ( 3, 2, 2, 2, 3 ),
 ( 0.8125000000000000000, 0.8194444444444444198, 0.8333333333333333703, 0.8472222222222222099, 0.8541666666666667407 ),
 .UNSPECIFIED. ) 
 CURVE ( )  GEOMETRIC_REPRESENTATION_ITEM ( )  RATIONAL_B_SPLINE_CURVE ( ( 0.9330127018922194093, 0.9330127018922194093, 1.000000000000000000, 0.8660254037844387076, 1.000000000000000000, 0.8660254037844387076, 1.000000000000000000, 0.9330127018922187432, 0.9330127018922192983 ) ) 
 REPRESENTATION_ITEM ( '' )  );
#4431=DIRECTION ( 'NONE',  ( 0.000000000000000000, 1.000000000000000000, 0.000000000000000000 ) ) ;
#4435=CARTESIAN_POINT ( 'NONE',  ( -27.24356964374999279, 196.6906250006145456, 15.72908226750539384 ) ) ;
#4451=CARTESIAN_POINT ( 'NONE',  ( -26.99999999999998934, 198.6875000000000284, 15.58845726811991561 ) ) ;
#4452=ORIENTED_EDGE ( 'NONE', *, *, #8939, .F. ) ;
#4454=ORIENTED_EDGE ( 'NONE', *, *, #35475, .T. ) ;
#4465=AXIS2_PLACEMENT_3D ( 'NONE', #37028, #37216, #2355 ) ;
#4483=CYLINDRICAL_SURFACE ( 'NONE', #15052, 25.00000000000000000 ) ;
#4509=ORIENTED_EDGE ( 'NONE', *, *, #18682, .T. ) ;
#4532=LINE ( 'NONE', #16293, #34504 ) ;
#4538=ORIENTED_EDGE ( 'NONE', *, *, #36547, .F. ) ;
#4560=CARTESIAN_POINT ( 'NONE',  ( 13.62178482187499640, 196.0531250006145285, -23.59362340125807123 ) ) ;
#4571=ORIENTED_EDGE ( 'NONE', *, *, #13873, .T. ) ;
#4573=CARTESIAN_POINT ( 'NONE',  ( 0.000000000000000000, 0.000000000000000000, 0.000000000000000000 ) ) ;
#4586=CARTESIAN_POINT ( 'NONE',  ( -27.24356964375000345, 197.1031250006145399, 0.000000000000000000 ) ) ;
#4608=CARTESIAN_POINT ( 'NONE',  ( 3.306546357697854128E-15, 200.0000000000000000, 27.00000000000000355 ) ) ;
#4620=ORIENTED_EDGE ( 'NONE', *, *, #20907, .T. ) ;
#4622=CARTESIAN_POINT ( 'NONE',  ( 5.778771075727756162E-15, 198.1156250006145285, 31.45816453501076637 ) ) ;
#4623=CARTESIAN_POINT ( 'NONE',  ( -27.24356964375000345, 199.4093750006145456, 0.000000000000000000 ) ) ;
#4636=CARTESIAN_POINT ( 'NONE',  ( 6.123233995736766282E-16, 2.000000000000000000, 5.000000000000000000 ) ) ;
#4637=CARTESIAN_POINT ( 'NONE',  ( -13.49999999999998401, 197.3750000000000284, 23.38268590217985476 ) ) ;
#4641=ORIENTED_EDGE ( 'NONE', *, *, #36536, .T. ) ;
#4651=DIRECTION ( 'NONE',  ( 0.000000000000000000, 0.000000000000000000, 1.000000000000000000 ) ) ;
#4715=CARTESIAN_POINT ( 'NONE',  ( -7.234628195640263826, 195.5200961906613770, -27.00000000000003553 ) ) ;
#4734=CARTESIAN_POINT ( 'NONE',  ( -27.24356964374999279, 194.9468750006145683, 15.72908226750539384 ) ) ;
#4748=CARTESIAN_POINT ( 'NONE',  ( 27.24356964375000345, 195.0781250006145342, -3.336375036156643733E-15 ) ) ;
#4759=DIRECTION ( 'NONE',  ( -0.000000000000000000, -1.000000000000000000, -0.000000000000000000 ) ) ;
#4771=CARTESIAN_POINT ( 'NONE',  ( 27.24356964374999635, 195.5656250006145171, -15.72908226750539029 ) ) ;
#4786=UNCERTAINTY_MEASURE_WITH_UNIT (LENGTH_MEASURE( 1.000000000000000082E-05 ), #19083, 'distance_accuracy_value', 'NONE');
#4808=CARTESIAN_POINT ( 'NONE',  ( 5.778771075727756162E-15, 198.1718750006145342, 31.45816453501075927 ) ) ;
#4811=CARTESIAN_POINT ( 'NONE',  ( -13.49999999999998401, 195.1250000000000284, 23.38268590217985476 ) ) ;
#4822=CARTESIAN_POINT ( 'NONE',  ( -13.50000000000000533, 196.7750000000000057, -23.38268590217984411 ) ) ;
#4914=LINE ( 'NONE', #5104, #2719 ) ;
#4926=VERTEX_POINT ( 'NONE', #24357 ) ;
#4927=CARTESIAN_POINT ( 'NONE',  ( 27.24356964375000700, 195.0406250006145399, 15.72908226750537075 ) ) ;
#4940=CARTESIAN_POINT ( 'NONE',  ( 1.255007937094097924E-14, 199.4375000000000284, -27.00000000000000000 ) ) ;
#4945=CARTESIAN_POINT ( 'NONE',  ( 0.000000000000000000, 200.0000000000000000, 0.000000000000000000 ) ) ;
#4947=VECTOR ( 'NONE', #1686, 1000.000000000000000 ) ;
#4949=CARTESIAN_POINT ( 'NONE',  ( -27.24356964375000345, 196.2031250006145342, 0.000000000000000000 ) ) ;
#4957=ORIENTED_EDGE ( 'NONE', *, *, #728, .F. ) ;
#4978=CARTESIAN_POINT ( 'NONE',  ( 13.49999999999999645, 195.9125000012290343, -23.38268590217984766 ) ) ;
#4989=CARTESIAN_POINT ( 'NONE',  ( 5.778771075727756162E-15, 195.4156250006145399, 31.45816453501076637 ) ) ;
#4991=CARTESIAN_POINT ( 'NONE',  ( 5.778771075727756162E-15, 199.0718750006145399, 31.45816453501075927 ) ) ;
#5009=CARTESIAN_POINT ( 'NONE',  ( -27.00000000000000355, 198.1625000000000227, -15.58845726811989429 ) ) ;
#5013=VERTEX_POINT ( 'NONE', #19056 ) ;
#5050=CARTESIAN_POINT ( 'NONE',  ( -4.694659320240884604E-14, 197.5250000012290172, 27.00000000000000000 ) ) ;
#5089=CARTESIAN_POINT ( 'NONE',  ( -27.00000000000000355, 195.6125000012290513, 0.000000000000000000 ) ) ;
#5091=CYLINDRICAL_SURFACE ( 'NONE', #14055, 27.00000000000000355 ) ;
#5104=CARTESIAN_POINT ( 'NONE',  ( 3.306546357697854128E-15, 200.0000000000000000, 27.00000000000000355 ) ) ;
#5106=CARTESIAN_POINT ( 'NONE',  ( -27.24356964375000345, 195.7718750006145569, -15.72908226750537786 ) ) ;
#5117=CARTESIAN_POINT ( 'NONE',  ( -13.62178482187498396, 194.9281250006145569, 23.59362340125808188 ) ) ;
#5138=CARTESIAN_POINT ( 'NONE',  ( -27.24356964374999635, 196.2406250006145285, 15.72908226750539384 ) ) ;
#5153=CARTESIAN_POINT ( 'NONE',  ( -13.50000000000000533, 199.9250000000000114, -23.38268590217984411 ) ) ;
#5165=CARTESIAN_POINT ( 'NONE',  ( 0.000000000000000000, 200.0000000000000000, 0.000000000000000000 ) ) ;
#5174=CARTESIAN_POINT ( 'NONE',  ( 0.000000000000000000, 0.000000000000000000, -27.00000000000000355 ) ) ;
#5175=ORIENTED_EDGE ( 'NONE', *, *, #15166, .T. ) ;
#5177=CIRCLE ( 'NONE', #17289, 5.000000000000000000 ) ;
#5178=CARTESIAN_POINT ( 'NONE',  ( -27.24356964374999279, 194.8906250006145342, 15.72908226750539384 ) ) ;
#5179=CARTESIAN_POINT ( 'NONE',  ( -27.24356964374999990, 198.9218750006145626, -15.72908226750537786 ) ) ;
#5182=ADVANCED_FACE ( 'NONE', ( #36646 ), #27566, .T. ) ;
#5183=CARTESIAN_POINT ( 'NONE',  ( 7.234628195640363302, 196.3799038117967086, -26.99999999999996803 ) ) ;
#5197=CARTESIAN_POINT ( 'NONE',  ( -27.00000000000000355, 195.0500000000000114, 0.000000000000000000 ) ) ;
#5222=ORIENTED_EDGE ( 'NONE', *, *, #15718, .T. ) ;
#5230=AXIS2_PLACEMENT_3D ( 'NONE', #5165, #5353, #37001 ) ;
#5238=CARTESIAN_POINT ( 'NONE',  ( 26.99999999999999645, 197.6750000012290229, -15.58845726811990495 ) ) ;
#5255=CARTESIAN_POINT ( 'NONE',  ( 0.000000000000000000, 200.0000000000000000, 0.000000000000000000 ) ) ;
#5276=CARTESIAN_POINT ( 'NONE',  ( -13.62178482187500528, 199.2781250006145228, -23.59362340125807123 ) ) ;
#5298=EDGE_CURVE ( 'NONE', #29410, #26583, #5658, .T. ) ;
#5303=CARTESIAN_POINT ( 'NONE',  ( 13.49999999999999645, 198.6125000012290513, -23.38268590217984766 ) ) ;
#5327=CARTESIAN_POINT ( 'NONE',  ( -13.62178482187498396, 195.3781250006145171, 23.59362340125808188 ) ) ;
#5353=DIRECTION ( 'NONE',  ( -0.000000000000000000, -1.000000000000000000, -0.000000000000000000 ) ) ;
#5362=CARTESIAN_POINT ( 'NONE',  ( 13.62178482187501416, 195.9031250006145513, 23.59362340125806767 ) ) ;
#5363=CARTESIAN_POINT ( 'NONE',  ( 27.24356964374999635, 199.2218750006145456, -15.72908226750539029 ) ) ;
#5365=PLANE ( 'NONE',  #35980 ) ;
#5377=CARTESIAN_POINT ( 'NONE',  ( 13.49999999999999645, 195.8000000000000114, -23.38268590217984766 ) ) ;
#5428=VERTEX_POINT ( 'NONE', #5733 ) ;
#5446=ORIENTED_EDGE ( 'NONE', *, *, #20976, .T. ) ;
#5449=CYLINDRICAL_SURFACE ( 'NONE', #30803, 27.00000000000000355 ) ;
#5476=CARTESIAN_POINT ( 'NONE',  ( -20.68320086892770604, 194.6619763917542798, -17.35526438333879540 ) ) ;
#5480=CARTESIAN_POINT ( 'NONE',  ( 27.00000000000001066, 198.0500000012290513, 15.58845726811988897 ) ) ;
#5499=CARTESIAN_POINT ( 'NONE',  ( 1.255007937094097924E-14, 199.4375000000000284, -27.00000000000000355 ) ) ;
#5529=VERTEX_POINT ( 'NONE', #8037 ) ;
#5530=CARTESIAN_POINT ( 'NONE',  ( -7.234628195640263826, 196.7575961894323484, -27.00000000000003553 ) ) ;
#5542=CARTESIAN_POINT ( 'NONE',  ( -27.24356964375000345, 194.8531250006145115, 0.000000000000000000 ) ) ;
#5543=CARTESIAN_POINT ( 'NONE',  ( -27.24356964374999990, 199.7656250006145342, -15.72908226750537786 ) ) ;
#5546=EDGE_CURVE ( 'NONE', #33961, #26752, #22404, .T. ) ;
#5562=CARTESIAN_POINT ( 'NONE',  ( -1.909035429704832693E-15, 195.3874999999999886, -31.17691453623979214 ) ) ;
#5568=FACE_OUTER_BOUND ( 'NONE', #9147, .T. ) ;
#5600=VERTEX_POINT ( 'NONE', #21295 ) ;
#5626=( BOUNDED_CURVE ( )  B_SPLINE_CURVE ( 2, ( #25808, #16551, #5153, #33971, #19221 ),
 .UNSPECIFIED., .F., .F. ) 
 B_SPLINE_CURVE_WITH_KNOTS ( ( 3, 2, 3 ),
 ( 0.000000000000000000, 0.01388888888888888985, 0.02083333333333333565 ),
 .UNSPECIFIED. ) 
 CURVE ( )  GEOMETRIC_REPRESENTATION_ITEM ( )  RATIONAL_B_SPLINE_CURVE ( ( 1.000000000000000000, 0.8660254037844387076, 1.000000000000000000, 0.9330127018922192983, 0.9330127018922194093 ) ) 
 REPRESENTATION_ITEM ( '' )  );
#5658=CIRCLE ( 'NONE', #15356, 25.00000000000000000 ) ;
#5668=CARTESIAN_POINT ( 'NONE',  ( -26.99999999999998934, 197.0000000012290400, 15.58845726811991561 ) ) ;
#5679=DIRECTION ( 'NONE',  ( 0.000000000000000000, -1.000000000000000000, 0.000000000000000000 ) ) ;
#5694=STYLED_ITEM ( 'NONE', ( #22290 ), #22840 ) ;
#5699=CARTESIAN_POINT ( 'NONE',  ( -27.24356964375000345, 198.9593750006145285, 0.000000000000000000 ) ) ;
#5707=EDGE_CURVE ( 'NONE', #10453, #29410, #9344, .T. ) ;
#5710=CARTESIAN_POINT ( 'NONE',  ( 13.62178482187501416, 199.5031250006145456, 23.59362340125806767 ) ) ;
#5715=ADVANCED_FACE ( 'NONE', ( #29993 ), #4024, .T. ) ;
#5727=( BOUNDED_CURVE ( )  B_SPLINE_CURVE ( 2, ( #15743, #1135, #10045, #21255, #1325, #32604, #21622, #18600, #26723 ),
 .UNSPECIFIED., .F., .F. ) 
 B_SPLINE_CURVE_WITH_KNOTS ( ( 3, 2, 2, 2, 3 ),
 ( 0.02083333333333333565, 0.02777777777777777624, 0.04166666666666666435, 0.05555555555555555247, 0.06250000000000000000 ),
 .UNSPECIFIED. ) 
 CURVE ( )  GEOMETRIC_REPRESENTATION_ITEM ( )  RATIONAL_B_SPLINE_CURVE ( ( 0.9330127018922194093, 0.9330127018922194093, 1.000000000000000000, 0.8660254037844387076, 1.000000000000000000, 0.8660254037844387076, 1.000000000000000000, 0.9330127018922194093, 0.9330127018922194093 ) ) 
 REPRESENTATION_ITEM ( '' )  );
#5731=CARTESIAN_POINT ( 'NONE',  ( -3.253724281355068545E-15, 198.6500000012290172, -27.00000000000000000 ) ) ;
#5732=CARTESIAN_POINT ( 'NONE',  ( 27.24356964375000700, 196.8968750006145285, 15.72908226750537075 ) ) ;
#5733=CARTESIAN_POINT ( 'NONE',  ( 5.438367727407757775E-14, 198.0875000000000057, -27.00000000000000355 ) ) ;
#5751=CARTESIAN_POINT ( 'NONE',  ( -13.62178482187498396, 199.0343750006145456, 23.59362340125808188 ) ) ;
#5775=VERTEX_POINT ( 'NONE', #4211 ) ;
#5776=LINE ( 'NONE', #28523, #7756 ) ;
#5792=ORIENTED_EDGE ( 'NONE', *, *, #36303, .F. ) ;
#5834=DIRECTION ( 'NONE',  ( -0.000000000000000000, -1.000000000000000000, -0.000000000000000000 ) ) ;
#5838=CARTESIAN_POINT ( 'NONE',  ( 27.00000000000001421, 198.5000000012290684, 15.58845726811988897 ) ) ;
#5839=ORIENTED_EDGE ( 'NONE', *, *, #36547, .T. ) ;
#5858=CARTESIAN_POINT ( 'NONE',  ( -13.50000000000000533, 196.8875000012290286, -23.38268590217984411 ) ) ;
#5888=CARTESIAN_POINT ( 'NONE',  ( -1.926257025242585782E-15, 199.7468750006145513, -31.45816453501076637 ) ) ;
#5919=CARTESIAN_POINT ( 'NONE',  ( 13.62178482187501416, 196.8593750006145342, 23.59362340125806767 ) ) ;
#5939=CARTESIAN_POINT ( 'NONE',  ( -27.24356964374999635, 197.1968750006145115, 15.72908226750539384 ) ) ;
#5958=DIRECTION ( 'NONE',  ( 0.8660254037844187236, -0.5000000000000346390, 0.000000000000000000 ) ) ;
#5962=DIRECTION ( 'NONE',  ( -0.6427875693915772182, 0.000000000000000000, 0.7660444769304640689 ) ) ;
#5980=LINE ( 'NONE', #12043, #8814 ) ;
#6041=CARTESIAN_POINT ( 'NONE',  ( -27.00000000000000355, 196.4750000012290343, -15.58845726811989429 ) ) ;
#6058=CARTESIAN_POINT ( 'NONE',  ( -27.24356964375000345, 194.8857344423842619, -9.915847606754343957 ) ) ;
#6061=CARTESIAN_POINT ( 'NONE',  ( 1.120210788295102201E-13, 195.5000000012290400, -27.00000000000000711 ) ) ;
#6070=CARTESIAN_POINT ( 'NONE',  ( -27.24356964375000345, 199.3718750006145513, -15.72908226750537786 ) ) ;
#6072=ORIENTED_EDGE ( 'NONE', *, *, #18466, .F. ) ;
#6074=VECTOR ( 'NONE', #305, 1000.000000000000000 ) ;
#6083=CARTESIAN_POINT ( 'NONE',  ( -27.24356964374999990, 199.3156250006145171, -15.72908226750537786 ) ) ;
#6105=CARTESIAN_POINT ( 'NONE',  ( -27.24356964375000345, 196.2593750006145399, 0.000000000000000000 ) ) ;
#6125=CARTESIAN_POINT ( 'NONE',  ( 27.24356964374999635, 198.7718750006145569, -15.72908226750539029 ) ) ;
#6127=ORIENTED_EDGE ( 'NONE', *, *, #12350, .T. ) ;
#6143=LINE ( 'NONE', #14316, #17394 ) ;
#6156=CARTESIAN_POINT ( 'NONE',  ( 5.778771075727756162E-15, 199.4656250006145797, 31.45816453501076637 ) ) ;
#6162=CYLINDRICAL_SURFACE ( 'NONE', #12988, 27.00000000000000355 ) ;
#6200=EDGE_CURVE ( 'NONE', #32805, #32692, #5177, .T. ) ;
#6214=CARTESIAN_POINT ( 'NONE',  ( 7.234628195640322446, 199.6825961894323598, 26.99999999999999645 ) ) ;
#6228=ORIENTED_EDGE ( 'NONE', *, *, #27306, .F. ) ;
#6237=CARTESIAN_POINT ( 'NONE',  ( -27.00000000000000355, 196.9625000012290172, 0.000000000000000000 ) ) ;
#6254=CYLINDRICAL_SURFACE ( 'NONE', #4320, 5.000000000000000000 ) ;
#6259=CARTESIAN_POINT ( 'NONE',  ( 13.62178482187499640, 196.1093750006145342, -23.59362340125807123 ) ) ;
#6266=PLANE ( 'NONE',  #10014 ) ;
#6270=CARTESIAN_POINT ( 'NONE',  ( 13.62178482187501416, 199.1093750006145342, 23.59362340125806767 ) ) ;
#6281=CARTESIAN_POINT ( 'NONE',  ( 27.24356964375000345, 198.6781250006145569, -3.336375036156643733E-15 ) ) ;
#6304=CARTESIAN_POINT ( 'NONE',  ( 1.069080835302379631E-14, 198.8750000012290400, 27.00000000000000000 ) ) ;
#6306=CARTESIAN_POINT ( 'NONE',  ( -1.926257025242585782E-15, 195.6968750006145683, -31.45816453501075927 ) ) ;
#6321=CARTESIAN_POINT ( 'NONE',  ( -13.62178482187498396, 198.5843750006145569, 23.59362340125808188 ) ) ;
#6350=CARTESIAN_POINT ( 'NONE',  ( 27.24356964375000345, 199.5781250006145342, -3.336375036156643733E-15 ) ) ;
#6366=LINE ( 'NONE', #32699, #16090 ) ;
#6390=ORIENTED_EDGE ( 'NONE', *, *, #20591, .T. ) ;
#6403=CARTESIAN_POINT ( 'NONE',  ( 27.00000000000001421, 199.7375000000000114, 15.58845726811988897 ) ) ;
#6426=VECTOR ( 'NONE', #4288, 1000.000000000000000 ) ;
#6427=CARTESIAN_POINT ( 'NONE',  ( -1.909035429704832693E-15, 197.7500000012290400, -31.17691453623979214 ) ) ;
#6447=CARTESIAN_POINT ( 'NONE',  ( -27.24356964375000345, 195.3593750006145342, 0.000000000000000000 ) ) ;
#6457=DIRECTION ( 'NONE',  ( 0.000000000000000000, 1.000000000000000000, 0.000000000000000000 ) ) ;
#6462=CARTESIAN_POINT ( 'NONE',  ( 27.24356964375000700, 198.6968750006145115, 15.72908226750537075 ) ) ;
#6472=ORIENTED_EDGE ( 'NONE', *, *, #25994, .F. ) ;
#6474=CARTESIAN_POINT ( 'NONE',  ( -13.62178482187498396, 198.9781250006145399, 23.59362340125808188 ) ) ;
#6479=AXIS2_PLACEMENT_3D ( 'NONE', #12815, #35363, #29496 ) ;
#6481=CARTESIAN_POINT ( 'NONE',  ( 13.49999999999999645, 197.1500000000000057, -23.38268590217984766 ) ) ;
#6496=CARTESIAN_POINT ( 'NONE',  ( 27.24356964375000345, 198.6781250006145569, -3.336375036156643733E-15 ) ) ;
#6510=CARTESIAN_POINT ( 'NONE',  ( 5.778771075727756162E-15, 197.7218750006145456, 31.45816453501075927 ) ) ;
#6511=ORIENTED_EDGE ( 'NONE', *, *, #34489, .F. ) ;
#6515=CARTESIAN_POINT ( 'NONE',  ( 1.069080835302379631E-14, 195.6124999999999829, 27.00000000000000000 ) ) ;
#6538=CARTESIAN_POINT ( 'NONE',  ( -27.24356964375000345, 199.8031250006145285, 0.000000000000000000 ) ) ;
#6554=CARTESIAN_POINT ( 'NONE',  ( -27.00000000000000355, 199.5500000000000114, 0.000000000000000000 ) ) ;
#6577=EDGE_LOOP ( 'NONE', ( #17723, #29316 ) ) ;
#6591=CARTESIAN_POINT ( 'NONE',  ( 3.253724281355069334E-15, 199.8875000000000455, -27.00000000000000000 ) ) ;
#6613=CARTESIAN_POINT ( 'NONE',  ( -13.49999999999998401, 195.2375000012290229, 23.38268590217985476 ) ) ;
#6630=CARTESIAN_POINT ( 'NONE',  ( -7.234628195640302017, 199.1924038105676686, 27.00000000000000711 ) ) ;
#6644=CARTESIAN_POINT ( 'NONE',  ( -20.80759054502876282, 194.7557263913445809, -17.45964060548497088 ) ) ;
#6646=CARTESIAN_POINT ( 'NONE',  ( -27.24356964374999279, 197.6468750006145285, 15.72908226750539384 ) ) ;
#6647=ORIENTED_EDGE ( 'NONE', *, *, #12890, .T. ) ;
#6658=CARTESIAN_POINT ( 'NONE',  ( 27.24356964375000345, 196.8781250006145171, -3.336375036156643733E-15 ) ) ;
#6663=LINE ( 'NONE', #30165, #51 ) ;
#6669=VECTOR ( 'NONE', #1497, 1000.000000000000000 ) ;
#6678=ORIENTED_EDGE ( 'NONE', *, *, #1060, .F. ) ;
#6685=CARTESIAN_POINT ( 'NONE',  ( -1.926257025242585782E-15, 199.2406250006145285, -31.45816453501075927 ) ) ;
#6699=CARTESIAN_POINT ( 'NONE',  ( 27.24356964375000345, 198.7343750006145626, -3.336375036156643733E-15 ) ) ;
#6718=CARTESIAN_POINT ( 'NONE',  ( -20.77649301497164913, 194.9291638889422700, -17.43354668227102167 ) ) ;
#6726=CARTESIAN_POINT ( 'NONE',  ( 5.778771075727756162E-15, 197.6656250006145399, 31.45816453501076637 ) ) ;
#6737=FACE_OUTER_BOUND ( 'NONE', #11257, .T. ) ;
#6741=CARTESIAN_POINT ( 'NONE',  ( 13.49999999999999645, 199.4000000000000341, -23.38268590217984766 ) ) ;
#6792=ORIENTED_EDGE ( 'NONE', *, *, #22356, .T. ) ;
#6800=CARTESIAN_POINT ( 'NONE',  ( -27.00000000000000355, 195.1250000012290400, -15.58845726811989429 ) ) ;
#6820=CARTESIAN_POINT ( 'NONE',  ( -20.86978606573367045, 194.8588513912095550, -17.51182790300216752 ) ) ;
#6832=CARTESIAN_POINT ( 'NONE',  ( -27.24356964375000345, 197.6093750006145342, 0.000000000000000000 ) ) ;
#6839=( BOUNDED_CURVE ( )  B_SPLINE_CURVE ( 2, ( #30124, #21421, #10217, #13067, #15917, #19142, #1492, #12685, #33155 ),
 .UNSPECIFIED., .F., .F. ) 
 B_SPLINE_CURVE_WITH_KNOTS ( ( 3, 2, 2, 2, 3 ),
 ( 0.6875000000000000000, 0.6944444444444444198, 0.7083333333333333703, 0.7222222222222222099, 0.7291666666666667407 ),
 .UNSPECIFIED. ) 
 CURVE ( )  GEOMETRIC_REPRESENTATION_ITEM ( )  RATIONAL_B_SPLINE_CURVE ( ( 0.9330127018922194093, 0.9330127018922194093, 1.000000000000000000, 0.8660254037844387076, 1.000000000000000000, 0.8660254037844387076, 1.000000000000000000, 0.9330127018922187432, 0.9330127018922192983 ) ) 
 REPRESENTATION_ITEM ( '' )  );
#6846=CARTESIAN_POINT ( 'NONE',  ( -1.926257025242585782E-15, 197.4406250006145740, -31.45816453501075927 ) ) ;
#6854=CARTESIAN_POINT ( 'NONE',  ( 1.120210788295102201E-13, 197.1875000000000568, -27.00000000000000711 ) ) ;
#6875=CARTESIAN_POINT ( 'NONE',  ( 27.24356964374999635, 198.2656250006145058, -15.72908226750539029 ) ) ;
#6913=CARTESIAN_POINT ( 'NONE',  ( 1.069080835302379631E-14, 198.3124999999999716, 27.00000000000000000 ) ) ;
#6920=CARTESIAN_POINT ( 'NONE',  ( 13.62178482187501416, 197.7031250006145342, 23.59362340125806767 ) ) ;
#6921=CARTESIAN_POINT ( 'NONE',  ( 13.62178482187499640, 199.7093750006145285, -23.59362340125807123 ) ) ;
#6948=CARTESIAN_POINT ( 'NONE',  ( -27.00000000000000355, 198.2750000012290172, -15.58845726811989429 ) ) ;
#6953=LINE ( 'NONE', #15666, #24840 ) ;
#6962=PRODUCT_CONTEXT ( 'NONE', #26974, 'mechanical' ) ;
#7037=CARTESIAN_POINT ( 'NONE',  ( 13.62178482187499640, 196.1093750006145342, -23.59362340125807123 ) ) ;
#7049=CARTESIAN_POINT ( 'NONE',  ( -1.926257025242585782E-15, 196.5406250006145399, -31.45816453501075927 ) ) ;
#7074=CARTESIAN_POINT ( 'NONE',  ( 13.62178482187501416, 199.5031250006145456, 23.59362340125806767 ) ) ;
#7091=EDGE_CURVE ( 'NONE', #33961, #5428, #5980, .T. ) ;
#7111=CARTESIAN_POINT ( 'NONE',  ( -27.24356964374999279, 197.1406250006145342, 15.72908226750539384 ) ) ;
#7126=CARTESIAN_POINT ( 'NONE',  ( -26.99999999999998934, 197.3375000000000057, 15.58845726811991561 ) ) ;
#7161=CARTESIAN_POINT ( 'NONE',  ( 0.000000000000000000, 200.0000000000000000, 0.000000000000000000 ) ) ;
#7167=CARTESIAN_POINT ( 'NONE',  ( -20.68320042480033294, 194.9291638889422700, -17.35526491262919535 ) ) ;
#7221=CARTESIAN_POINT ( 'NONE',  ( 27.24356964374999279, 197.8718750006145513, -15.72908226750539207 ) ) ;
#7232=CARTESIAN_POINT ( 'NONE',  ( -27.24356964374999635, 196.6906250006145456, 15.72908226750539384 ) ) ;
#7254=CARTESIAN_POINT ( 'NONE',  ( -27.24356964374999990, 197.9656250006145228, -15.72908226750537786 ) ) ;
#7288=CARTESIAN_POINT ( 'NONE',  ( -13.50000000000000533, 197.3375000012290457, -23.38268590217984411 ) ) ;
#7291=CARTESIAN_POINT ( 'NONE',  ( -13.62178482187500528, 198.3781250006145171, -23.59362340125807123 ) ) ;
#7308=CARTESIAN_POINT ( 'NONE',  ( -26.99999999999998934, 196.8875000000000171, 15.58845726811991561 ) ) ;
#7316=CARTESIAN_POINT ( 'NONE',  ( -7.234628195640354420, 196.4924038105676800, 26.99999999999996803 ) ) ;
#7391=EDGE_LOOP ( 'NONE', ( #33138, #6647, #18909, #8193 ) ) ;
#7400=CARTESIAN_POINT ( 'NONE',  ( 27.24356964375000345, 196.9343750006145228, -3.336375036156643733E-15 ) ) ;
#7411=ORIENTED_EDGE ( 'NONE', *, *, #16798, .T. ) ;
#7413=ADVANCED_FACE ( 'NONE', ( #6737 ), #18311, .T. ) ;
#7415=CARTESIAN_POINT ( 'NONE',  ( 13.62178482187499640, 196.9531250006145342, -23.59362340125807123 ) ) ;
#7429=CARTESIAN_POINT ( 'NONE',  ( 27.00000000000001421, 195.3500000012290343, 15.58845726811988897 ) ) ;
#7432=CARTESIAN_POINT ( 'NONE',  ( 1.069080835302379631E-14, 199.2125000000000057, 27.00000000000000000 ) ) ;
#7439=CARTESIAN_POINT ( 'NONE',  ( -27.24356964374999635, 195.7906250006145115, 15.72908226750539384 ) ) ;
#7452=MANIFOLD_SOLID_BREP ( 'Thread1', #29547 ) ;
#7463=LINE ( 'NONE', #4608, #20972 ) ;
#7475=CARTESIAN_POINT ( 'NONE',  ( 13.62178482187501416, 198.1531250006145228, 23.59362340125806767 ) ) ;
#7480=AXIS2_PLACEMENT_3D ( 'NONE', #13535, #10684, #1595 ) ;
#7486=( LENGTH_UNIT ( ) NAMED_UNIT ( * ) SI_UNIT ( .MILLI., .METRE. ) );
#7492=CARTESIAN_POINT ( 'NONE',  ( 27.00000000000001066, 197.4875000000000114, 15.58845726811988897 ) ) ;
#7501=CARTESIAN_POINT ( 'NONE',  ( 3.306546357697854128E-15, 200.0000000000000000, 27.00000000000000355 ) ) ;
#7590=CARTESIAN_POINT ( 'NONE',  ( 27.24356964375000700, 195.0968750006145456, 15.72908226750537075 ) ) ;
#7601=CARTESIAN_POINT ( 'NONE',  ( -1.909035429704832693E-15, 199.1000000012290627, -31.17691453623979214 ) ) ;
#7613=CARTESIAN_POINT ( 'NONE',  ( 1.120210788295102201E-13, 195.0500000012290798, -27.00000000000000711 ) ) ;
#7625=EDGE_CURVE ( 'NONE', #32085, #33186, #15648, .T. ) ;
#7626=CARTESIAN_POINT ( 'NONE',  ( -1.926257025242585782E-15, 195.6406250006145058, -31.45816453501075927 ) ) ;
#7665=CARTESIAN_POINT ( 'NONE',  ( 27.24356964374999279, 195.1156250006145285, -15.72908226750539207 ) ) ;
#7666=CARTESIAN_POINT ( 'NONE',  ( -27.24356964375000345, 198.0593750006145513, 0.000000000000000000 ) ) ;
#7669=FACE_OUTER_BOUND ( 'NONE', #23163, .T. ) ;
#7680=CARTESIAN_POINT ( 'NONE',  ( -27.00000000000000355, 198.6125000000000398, -15.58845726811989429 ) ) ;
#7756=VECTOR ( 'NONE', #11649, 1000.000000000000000 ) ;
#7776=CARTESIAN_POINT ( 'NONE',  ( 13.62178482187499640, 195.2093750006145569, -23.59362340125807123 ) ) ;
#7783=CYLINDRICAL_SURFACE ( 'NONE', #11933, 27.00000000000000355 ) ;
#7788=CARTESIAN_POINT ( 'NONE',  ( 26.99999999999999645, 198.1250000012290400, -15.58845726811990495 ) ) ;
#7794=EDGE_CURVE ( 'NONE', #17216, #5013, #27491, .T. ) ;
#7801=CARTESIAN_POINT ( 'NONE',  ( -13.49999999999998401, 195.2375000012290229, 23.38268590217985476 ) ) ;
#7813=CARTESIAN_POINT ( 'NONE',  ( -27.24356964374999635, 195.3406250006145513, 15.72908226750539384 ) ) ;
#7850=CARTESIAN_POINT ( 'NONE',  ( 5.778771075727756162E-15, 195.8656250006145285, 31.45816453501076637 ) ) ;
#7851=CARTESIAN_POINT ( 'NONE',  ( -1.926257025242585782E-15, 199.2968750006145342, -31.45816453501075927 ) ) ;
#7867=CARTESIAN_POINT ( 'NONE',  ( 5.727106289114498080E-15, 196.9625000000000057, 31.17691453623979214 ) ) ;
#7948=CARTESIAN_POINT ( 'NONE',  ( -7.234628195640328663, 197.3924038105676857, 26.99999999999999289 ) ) ;
#7972=CARTESIAN_POINT ( 'NONE',  ( 13.62178482187501416, 195.0031250006145456, 23.59362340125806767 ) ) ;
#7994=VECTOR ( 'NONE', #5834, 1000.000000000000000 ) ;
#7996=CARTESIAN_POINT ( 'NONE',  ( 27.24356964375000345, 196.4281250006145569, -3.336375036156643733E-15 ) ) ;
#8032=CARTESIAN_POINT ( 'NONE',  ( 7.234628195640269155, 194.8450961906613941, 27.00000000000003197 ) ) ;
#8035=CARTESIAN_POINT ( 'NONE',  ( 13.62178482187499640, 196.0531250006145285, -23.59362340125807123 ) ) ;
#8036=CARTESIAN_POINT ( 'NONE',  ( -13.62178482187498396, 199.4843750006145626, 23.59362340125808188 ) ) ;
#8037=CARTESIAN_POINT ( 'NONE',  ( -27.24356964375000345, 199.8593750006145342, 0.000000000000000000 ) ) ;
#8053=CARTESIAN_POINT ( 'NONE',  ( -27.00000000000000355, 196.4000000000000057, 0.000000000000000000 ) ) ;
#8091=ADVANCED_FACE ( 'NONE', ( #29363 ), #25778, .F. ) ;
#8100=ORIENTED_EDGE ( 'NONE', *, *, #17818, .F. ) ;
#8115=DIRECTION ( 'NONE',  ( 0.000000000000000000, 1.000000000000000000, 0.000000000000000000 ) ) ;
#8139=DIRECTION ( 'NONE',  ( 0.000000000000000000, 0.000000000000000000, -1.000000000000000000 ) ) ;
#8164=CARTESIAN_POINT ( 'NONE',  ( -27.00000000000000355, 199.6625000012290343, 0.000000000000000000 ) ) ;
#8178=CARTESIAN_POINT ( 'NONE',  ( 27.00000000000000355, 197.9750000000000227, -3.306546357697854128E-15 ) ) ;
#8186=CARTESIAN_POINT ( 'NONE',  ( -13.62178482187500528, 196.5781250006145342, -23.59362340125807123 ) ) ;
#8193=ORIENTED_EDGE ( 'NONE', *, *, #34880, .F. ) ;
#8224=CARTESIAN_POINT ( 'NONE',  ( -13.62178482187500528, 195.2281250006145399, -23.59362340125807123 ) ) ;
#8225=CARTESIAN_POINT ( 'NONE',  ( 27.24356964375000345, 197.8343750006145569, -3.336375036156643733E-15 ) ) ;
#8242=CARTESIAN_POINT ( 'NONE',  ( 13.62178482187501416, 199.5593750006145513, 23.59362340125806767 ) ) ;
#8293=ORIENTED_EDGE ( 'NONE', *, *, #13054, .F. ) ;
#8322=EDGE_CURVE ( 'NONE', #2775, #1851, #21471, .T. ) ;
#8346=CARTESIAN_POINT ( 'NONE',  ( 5.727106289114498080E-15, 199.3250000012290570, 31.17691453623979214 ) ) ;
#8359=AXIS2_PLACEMENT_3D ( 'NONE', #34142, #22224, #1744 ) ;
#8367=FACE_OUTER_BOUND ( 'NONE', #17324, .T. ) ;
#8370=CARTESIAN_POINT ( 'NONE',  ( -13.62178482187498396, 194.9281250006145569, 23.59362340125808188 ) ) ;
#8371=CARTESIAN_POINT ( 'NONE',  ( 0.000000000000000000, 2.000000000000000000, 0.000000000000000000 ) ) ;
#8376=CIRCLE ( 'NONE', #34985, 27.00000000000000355 ) ;
#8408=CARTESIAN_POINT ( 'NONE',  ( -20.86978604919638869, 194.8588513911398081, -17.51182792271053046 ) ) ;
#8418=ORIENTED_EDGE ( 'NONE', *, *, #18682, .F. ) ;
#8423=CARTESIAN_POINT ( 'NONE',  ( 5.778771075727756162E-15, 199.5218750006145854, 31.45816453501075927 ) ) ;
#8500=CARTESIAN_POINT ( 'NONE',  ( -26.99999999999999645, 197.0000000012290116, 15.58845726811991561 ) ) ;
#8528=CARTESIAN_POINT ( 'NONE',  ( 13.50000000000001421, 196.2125000012290172, 23.38268590217984055 ) ) ;
#8558=( BOUNDED_CURVE ( )  B_SPLINE_CURVE ( 2, ( #10125, #10491, #18677, #13530, #24900, #33248, #7288, #1209, #27561 ),
 .UNSPECIFIED., .F., .F. ) 
 B_SPLINE_CURVE_WITH_KNOTS ( ( 3, 2, 2, 2, 3 ),
 ( 0.3958333333333333703, 0.4027777777777777901, 0.4166666666666666852, 0.4305555555555555802, 0.4375000000000000000 ),
 .UNSPECIFIED. ) 
 CURVE ( )  GEOMETRIC_REPRESENTATION_ITEM ( )  RATIONAL_B_SPLINE_CURVE ( ( 0.9330127018922194093, 0.9330127018922196314, 1.000000000000000000, 0.8660254037844387076, 1.000000000000000000, 0.8660254037844387076, 1.000000000000000000, 0.9330127018922194093, 0.9330127018922194093 ) ) 
 REPRESENTATION_ITEM ( '' )  );
#8564=ADVANCED_FACE ( 'NONE', ( #32125 ), #6162, .T. ) ;
#8567=CARTESIAN_POINT ( 'NONE',  ( -27.24356964375000345, 199.8031250006145285, 0.000000000000000000 ) ) ;
#8570=FACE_OUTER_BOUND ( 'NONE', #34385, .T. ) ;
#8576=CARTESIAN_POINT ( 'NONE',  ( -27.24356964375000345, 199.8312500006145171, 0.000000000000000000 ) ) ;
#8586=CARTESIAN_POINT ( 'NONE',  ( 27.24356964375000345, 196.9343750006145228, -3.336375036156643733E-15 ) ) ;
#8589=CARTESIAN_POINT ( 'NONE',  ( -27.00000000000000355, 195.0500000000000114, 0.000000000000000000 ) ) ;
#8602=( BOUNDED_CURVE ( )  B_SPLINE_CURVE ( 2, ( #21794, #10220, #15729, #22352, #30316, #18956, #33901, #27658, #27279 ),
 .UNSPECIFIED., .F., .F. ) 
 B_SPLINE_CURVE_WITH_KNOTS ( ( 3, 2, 2, 2, 3 ),
 ( 0.3958333333333333703, 0.4027777777777777901, 0.4166666666666666852, 0.4305555555555555802, 0.4375000000000000000 ),
 .UNSPECIFIED. ) 
 CURVE ( )  GEOMETRIC_REPRESENTATION_ITEM ( )  RATIONAL_B_SPLINE_CURVE ( ( 0.9330127018922194093, 0.9330127018922196314, 1.000000000000000000, 0.8660254037844387076, 1.000000000000000000, 0.8660254037844387076, 1.000000000000000000, 0.9330127018922194093, 0.9330127018922194093 ) ) 
 REPRESENTATION_ITEM ( '' )  );
#8605=CARTESIAN_POINT ( 'NONE',  ( 27.24356964375000700, 199.1468750006145285, 15.72908226750537075 ) ) ;
#8618=( NAMED_UNIT ( * ) SI_UNIT ( $, .STERADIAN. ) SOLID_ANGLE_UNIT ( ) );
#8711=CARTESIAN_POINT ( 'NONE',  ( -26.99999999999998934, 195.6500000012290457, 15.58845726811991561 ) ) ;
#8730=VERTEX_POINT ( 'NONE', #4253 ) ;
#8753=CARTESIAN_POINT ( 'NONE',  ( 27.24356964375000700, 199.5406250006145683, 15.72908226750537075 ) ) ;
#8775=CARTESIAN_POINT ( 'NONE',  ( 13.62178482187499640, 195.6593750006145456, -23.59362340125807123 ) ) ;
#8794=CARTESIAN_POINT ( 'NONE',  ( 13.62178482187499640, 199.7093750006145285, -23.59362340125807123 ) ) ;
#8814=VECTOR ( 'NONE', #19858, 1000.000000000000000 ) ;
#8822=CARTESIAN_POINT ( 'NONE',  ( -27.00000000000000355, 194.6888594429640875, -9.827195528215911580 ) ) ;
#8830=CARTESIAN_POINT ( 'NONE',  ( -7.234628195640302017, 197.9549038117966973, 27.00000000000000711 ) ) ;
#8885=EDGE_LOOP ( 'NONE', ( #27251, #28943 ) ) ;
#8893=CARTESIAN_POINT ( 'NONE',  ( -13.49999999999998401, 197.4875000012290229, 23.38268590217985476 ) ) ;
#8911=CARTESIAN_POINT ( 'NONE',  ( 1.069080835302379631E-14, 196.6250000012290400, 27.00000000000000000 ) ) ;
#8914=CARTESIAN_POINT ( 'NONE',  ( -13.62178482187498396, 194.9843750006145626, 23.59362340125808188 ) ) ;
#8938=CARTESIAN_POINT ( 'NONE',  ( -27.24356964375000345, 199.3531250006145399, 0.000000000000000000 ) ) ;
#8939=EDGE_CURVE ( 'NONE', #5013, #36517, #22190, .T. ) ;
#8941=ADVANCED_FACE ( 'NONE', ( #25281 ), #37201, .T. ) ;
#8950=CARTESIAN_POINT ( 'NONE',  ( -20.80759054502876282, 194.9057263910046913, -17.45964060548497443 ) ) ;
#8951=ORIENTED_EDGE ( 'NONE', *, *, #29804, .F. ) ;
#8955=ADVANCED_FACE ( 'NONE', ( #22636, #7669 ), #5365, .F. ) ;
#8962=CARTESIAN_POINT ( 'NONE',  ( -1.926257025242585782E-15, 197.0468750006145626, -31.45816453501075927 ) ) ;
#8964=CARTESIAN_POINT ( 'NONE',  ( 1.069080835302379631E-14, 198.7624999999999886, 27.00000000000000000 ) ) ;
#8979=CARTESIAN_POINT ( 'NONE',  ( -27.24356964375000345, 197.1593750006145456, 0.000000000000000000 ) ) ;
#9007=CARTESIAN_POINT ( 'NONE',  ( -1.926257025242585782E-15, 199.6906250006145456, -31.45816453501076637 ) ) ;
#9025=CARTESIAN_POINT ( 'NONE',  ( 13.49999999999999645, 198.9500000000000171, -23.38268590217984766 ) ) ;
#9064=CARTESIAN_POINT ( 'NONE',  ( 27.00000000000000355, 198.5375000012290627, -3.306546357697854128E-15 ) ) ;
#9071=CARTESIAN_POINT ( 'NONE',  ( 7.234628195640363302, 196.7174038105676459, -26.99999999999996803 ) ) ;
#9086=CARTESIAN_POINT ( 'NONE',  ( 13.50000000000001421, 195.7625000012290570, 23.38268590217984055 ) ) ;
#9102=CARTESIAN_POINT ( 'NONE',  ( 7.234628195640363302, 195.0299038117966575, -26.99999999999996803 ) ) ;
#9120=ORIENTED_EDGE ( 'NONE', *, *, #20907, .F. ) ;
#9130=CARTESIAN_POINT ( 'NONE',  ( 5.778771075727756162E-15, 198.1156250006145285, 31.45816453501075927 ) ) ;
#9132=EDGE_CURVE ( 'NONE', #8730, #18034, #29922, .T. ) ;
#9147=EDGE_LOOP ( 'NONE', ( #2489, #6792, #34926, #17521 ) ) ;
#9151=CARTESIAN_POINT ( 'NONE',  ( -13.62178482187500528, 196.6343750006145399, -23.59362340125807123 ) ) ;
#9168=CARTESIAN_POINT ( 'NONE',  ( 27.24356964375000700, 198.2468750006145513, 15.72908226750537075 ) ) ;
#9208=CARTESIAN_POINT ( 'NONE',  ( 7.234628195640295800, 197.4325961894323882, 27.00000000000001066 ) ) ;
#9212=CARTESIAN_POINT ( 'NONE',  ( 27.00000000000001066, 198.8374999999999773, 15.58845726811988897 ) ) ;
#9214=ORIENTED_EDGE ( 'NONE', *, *, #728, .T. ) ;
#9251=CARTESIAN_POINT ( 'NONE',  ( 0.000000000000000000, 200.0000000000000000, -27.00000000000000355 ) ) ;
#9274=CARTESIAN_POINT ( 'NONE',  ( 27.00000000000000355, 197.6375000012290286, -3.306546357697854128E-15 ) ) ;
#9277=( BOUNDED_CURVE ( )  B_SPLINE_CURVE ( 2, ( #14789, #25782, #31841, #2081, #23139, #22955, #34870, #17451, #8911 ),
 .UNSPECIFIED., .F., .F. ) 
 B_SPLINE_CURVE_WITH_KNOTS ( ( 3, 2, 2, 2, 3 ),
 ( 0.5208333333333333703, 0.5277777777777777901, 0.5416666666666666297, 0.5555555555555555802, 0.5625000000000000000 ),
 .UNSPECIFIED. ) 
 CURVE ( )  GEOMETRIC_REPRESENTATION_ITEM ( )  RATIONAL_B_SPLINE_CURVE ( ( 0.9330127018922192983, 0.9330127018922198534, 1.000000000000000000, 0.8660254037844387076, 1.000000000000000000, 0.8660254037844387076, 1.000000000000000000, 0.9330127018922194093, 0.9330127018922194093 ) ) 
 REPRESENTATION_ITEM ( '' )  );
#9293=( BOUNDED_CURVE ( )  B_SPLINE_CURVE ( 2, ( #13680, #21648, #7801, #21835, #30555, #24487, #36217, #30170, #7613 ),
 .UNSPECIFIED., .F., .F. ) 
 B_SPLINE_CURVE_WITH_KNOTS ( ( 3, 2, 2, 2, 3 ),
 ( 0.8125000000000000000, 0.8194444444444444198, 0.8333333333333333703, 0.8472222222222222099, 0.8541666666666667407 ),
 .UNSPECIFIED. ) 
 CURVE ( )  GEOMETRIC_REPRESENTATION_ITEM ( )  RATIONAL_B_SPLINE_CURVE ( ( 0.9330127018922194093, 0.9330127018922194093, 1.000000000000000000, 0.8660254037844387076, 1.000000000000000000, 0.8660254037844387076, 1.000000000000000000, 0.9330127018922187432, 0.9330127018922192983 ) ) 
 REPRESENTATION_ITEM ( '' )  );
#9296=CARTESIAN_POINT ( 'NONE',  ( 13.62178482187501416, 196.8593750006145342, 23.59362340125806767 ) ) ;
#9305=CARTESIAN_POINT ( 'NONE',  ( -20.86978604919638869, 194.8026013911397456, -17.51182792271053046 ) ) ;
#9307=CARTESIAN_POINT ( 'NONE',  ( 13.62178482187499640, 198.8093750006145513, -23.59362340125807123 ) ) ;
#9318=CARTESIAN_POINT ( 'NONE',  ( 27.24356964375000345, 197.7781250006145228, -3.336375036156643733E-15 ) ) ;
#9343=CARTESIAN_POINT ( 'NONE',  ( 5.778771075727756162E-15, 198.1156250006145285, 31.45816453501075927 ) ) ;
#9344=LINE ( 'NONE', #15412, #18395 ) ;
#9350=ORIENTED_EDGE ( 'NONE', *, *, #12350, .F. ) ;
#9357=CARTESIAN_POINT ( 'NONE',  ( 13.62178482187501416, 198.6593750006145456, 23.59362340125806767 ) ) ;
#9380=DIRECTION ( 'NONE',  ( 1.000000000000000000, 0.000000000000000000, 0.000000000000000000 ) ) ;
#9425=ORIENTED_EDGE ( 'NONE', *, *, #1060, .T. ) ;
#9437=CARTESIAN_POINT ( 'NONE',  ( 13.50000000000001421, 198.4625000012290172, 23.38268590217984055 ) ) ;
#9481=CARTESIAN_POINT ( 'NONE',  ( 13.62178482187501416, 195.5093750006145399, 23.59362340125806767 ) ) ;
#9486=AXIS2_PLACEMENT_3D ( 'NONE', #18142, #32340, #23635 ) ;
#9491=DIRECTION ( 'NONE',  ( -0.000000000000000000, -1.000000000000000000, -0.000000000000000000 ) ) ;
#9493=CARTESIAN_POINT ( 'NONE',  ( 13.62178482187501416, 198.2093750006145285, 23.59362340125806767 ) ) ;
#9503=DIRECTION ( 'NONE',  ( 0.000000000000000000, -1.000000000000000000, 0.000000000000000000 ) ) ;
#9507=CARTESIAN_POINT ( 'NONE',  ( -13.62178482187500528, 197.0281250006145228, -23.59362340125807123 ) ) ;
#9530=CARTESIAN_POINT ( 'NONE',  ( -27.24356964374999635, 197.5906250006145228, 15.72908226750539384 ) ) ;
#9545=CARTESIAN_POINT ( 'NONE',  ( 27.24356964374999635, 196.9718750006145456, -15.72908226750539029 ) ) ;
#9546=VERTEX_POINT ( 'NONE', #36751 ) ;
#9570=CARTESIAN_POINT ( 'NONE',  ( 27.24356964375000345, 196.4281250006145569, -3.336375036156643733E-15 ) ) ;
#9587=FACE_OUTER_BOUND ( 'NONE', #33645, .T. ) ;
#9666=CARTESIAN_POINT ( 'NONE',  ( 1.069080835302379631E-14, 198.8750000012290400, 27.00000000000000000 ) ) ;
#9668=CARTESIAN_POINT ( 'NONE',  ( 27.24356964375000345, 196.0343750006145456, -3.336375036156643733E-15 ) ) ;
#9680=CARTESIAN_POINT ( 'NONE',  ( -27.24356964375000345, 196.2593750006145399, 0.000000000000000000 ) ) ;
#9688=CARTESIAN_POINT ( 'NONE',  ( -13.50000000000000533, 199.5875000012290457, -23.38268590217984411 ) ) ;
#9693=CARTESIAN_POINT ( 'NONE',  ( -13.62178482187500528, 195.6781250006145569, -23.59362340125807123 ) ) ;
#9709=EDGE_CURVE ( 'NONE', #32329, #25286, #27872, .T. ) ;
#9720=CARTESIAN_POINT ( 'NONE',  ( -13.62178482187498396, 198.5281250006145228, 23.59362340125808188 ) ) ;
#9722=CARTESIAN_POINT ( 'NONE',  ( 13.49999999999999645, 198.1625000012290343, -23.38268590217984766 ) ) ;
#9759=CARTESIAN_POINT ( 'NONE',  ( -13.62178482187500528, 197.4781250006145399, -23.59362340125807123 ) ) ;
#9863=CARTESIAN_POINT ( 'NONE',  ( -13.62178482187500528, 196.1843750006145228, -23.59362340125807123 ) ) ;
#9876=CARTESIAN_POINT ( 'NONE',  ( -13.62178482187500528, 196.1281250006145171, -23.59362340125807123 ) ) ;
#9891=CARTESIAN_POINT ( 'NONE',  ( -20.68320042480036491, 194.9994763866750134, -17.35526491262920246 ) ) ;
#9899=CARTESIAN_POINT ( 'NONE',  ( 27.24356964374999635, 199.1656250006145399, -15.72908226750539029 ) ) ;
#9925=VECTOR ( 'NONE', #11328, 1000.000000000000000 ) ;
#9940=CARTESIAN_POINT ( 'NONE',  ( -27.24356964375000345, 197.5156250006145342, -15.72908226750537786 ) ) ;
#9941=CARTESIAN_POINT ( 'NONE',  ( -13.62178482187500528, 199.7843750006145456, -23.59362340125807123 ) ) ;
#9956=CARTESIAN_POINT ( 'NONE',  ( -13.49999999999998401, 196.9250000000000114, 23.38268590217985476 ) ) ;
#9983=CARTESIAN_POINT ( 'NONE',  ( -27.00000000000000355, 196.0625000012290400, 0.000000000000000000 ) ) ;
#10014=AXIS2_PLACEMENT_3D ( 'NONE', #18599, #6457, #18029 ) ;
#10045=CARTESIAN_POINT ( 'NONE',  ( 13.49999999999999645, 199.5125000012290286, -23.38268590217984766 ) ) ;
#10050=CARTESIAN_POINT ( 'NONE',  ( -13.62178482187498396, 197.6843750006145228, 23.59362340125808188 ) ) ;
#10062=CARTESIAN_POINT ( 'NONE',  ( -27.24356964374999990, 195.2656250006145342, -15.72908226750537786 ) ) ;
#10078=CARTESIAN_POINT ( 'NONE',  ( 26.99999999999999645, 195.4250000012290229, -15.58845726811990495 ) ) ;
#10091=CARTESIAN_POINT ( 'NONE',  ( 27.24356964374999635, 199.6156250006145285, -15.72908226750539029 ) ) ;
#10125=CARTESIAN_POINT ( 'NONE',  ( -4.694659320240884604E-14, 197.5250000012290172, 27.00000000000000000 ) ) ;
#10129=CARTESIAN_POINT ( 'NONE',  ( -1.926257025242585782E-15, 197.4406250006145740, -31.45816453501076637 ) ) ;
#10130=CARTESIAN_POINT ( 'NONE',  ( 3.306546357697854128E-15, 200.0000000000000000, 27.00000000000000355 ) ) ;
#10144=DIRECTION ( 'NONE',  ( -0.000000000000000000, -1.000000000000000000, -0.000000000000000000 ) ) ;
#10145=CARTESIAN_POINT ( 'NONE',  ( 27.00000000000000355, 197.0749999999999886, -3.306546357697854128E-15 ) ) ;
#10150=DIRECTION ( 'NONE',  ( -0.000000000000000000, -1.000000000000000000, -0.000000000000000000 ) ) ;
#10152=CARTESIAN_POINT ( 'NONE',  ( -13.49999999999998401, 199.2875000012290627, 23.38268590217985476 ) ) ;
#10167=VECTOR ( 'NONE', #1177, 1000.000000000000000 ) ;
#10170=VERTEX_POINT ( 'NONE', #5476 ) ;
#10217=CARTESIAN_POINT ( 'NONE',  ( 13.49999999999999645, 196.2500000000000000, -23.38268590217984766 ) ) ;
#10220=CARTESIAN_POINT ( 'NONE',  ( -7.234628195640328663, 197.8424038105676743, 26.99999999999999289 ) ) ;
#10236=CARTESIAN_POINT ( 'NONE',  ( -27.24356964374999279, 196.7468750006145513, 15.72908226750539384 ) ) ;
#10248=CARTESIAN_POINT ( 'NONE',  ( 27.24356964375000700, 196.3906250006145058, 15.72908226750537075 ) ) ;
#10269=FACE_OUTER_BOUND ( 'NONE', #29814, .T. ) ;
#10273=CARTESIAN_POINT ( 'NONE',  ( 27.24356964375000345, 195.9781250006145399, -3.336375036156643733E-15 ) ) ;
#10312=CARTESIAN_POINT ( 'NONE',  ( -27.24356964374999279, 198.0406250006145399, 15.72908226750539384 ) ) ;
#10330=CYLINDRICAL_SURFACE ( 'NONE', #32926, 27.00000000000000355 ) ;
#10331=CARTESIAN_POINT ( 'NONE',  ( 5.727106289114498080E-15, 197.8625000000000114, 31.17691453623979214 ) ) ;
#10338=CARTESIAN_POINT ( 'NONE',  ( -27.00000000000000355, 199.1750000012290513, -15.58845726811989429 ) ) ;
#10351=VECTOR ( 'NONE', #2464, 1000.000000000000000 ) ;
#10410=CARTESIAN_POINT ( 'NONE',  ( -26.99999999999999645, 195.6500000012290457, 15.58845726811991561 ) ) ;
#10425=CARTESIAN_POINT ( 'NONE',  ( 13.62178482187501416, 195.0593750006145513, 23.59362340125806767 ) ) ;
#10437=CARTESIAN_POINT ( 'NONE',  ( -27.24356964375000345, 194.8531250006145115, 0.000000000000000000 ) ) ;
#10453=VERTEX_POINT ( 'NONE', #12764 ) ;
#10457=CARTESIAN_POINT ( 'NONE',  ( -13.62178482187500528, 195.6781250006145569, -23.59362340125807123 ) ) ;
#10491=CARTESIAN_POINT ( 'NONE',  ( -7.234628195640328663, 197.5049038117967086, 26.99999999999999289 ) ) ;
#10494=CARTESIAN_POINT ( 'NONE',  ( -27.24356964374999279, 195.7906250006145399, 15.72908226750539384 ) ) ;
#10495=CARTESIAN_POINT ( 'NONE',  ( -13.62178482187498396, 197.2343750006145626, 23.59362340125808188 ) ) ;
#10498=CARTESIAN_POINT ( 'NONE',  ( 27.00000000000000355, 195.7250000000000227, -3.306546357697854128E-15 ) ) ;
#10500=( BOUNDED_SURFACE ( )  B_SPLINE_SURFACE ( 1, 2, ( 
 ( #8567, #3245, #20888, #17290, #29012, #22978, #14439, #8753, #5710, #26740, #34706, #32429, #8938, #6083, #23, #580, #20134, #214, #17668, #25993, #18045, #17856, #6474, #11589, #29204, #14626, #14819, #20515, #32053, #28831, #6281, #32241, #23725, #26363, #31680, #2866, #398, #17479, #31865, #23534, #3056, #26177, #11964, #23165, #35080, #9130, #20696, #29398, #3432, #15000, #3624, #11779, #26552, #35263, #9318, #29587, #15192, #774, #15382, #15570, #32997, #32621, #15761, #6846, #21083, #12342, #13098, #30348, #27504, #18805, #4372, #15951, #1525, #21637, #9507, #3806, #7415, #27311, #6658, #24653, #18986, #36204, #35835, #7232, #1341, #12912, #18233, #7049, #12721, #24102, #24476, #10248, #21824, #35647, #33376, #26932, #962, #30543, #9876, #33189, #4560, #3996, #4188, #16135, #27126, #12538, #27687, #23916, #1151, #29775, #9693, #21269, #32807, #35457, #21457, #18617, #36022, #18423, #29967, #24291, #30159, #10062, #22382, #33931, #25023, #22566, #4748, #4927, #7972, #22010, #5117, #33748, #10437, #1714, #2458 ),
 ( #8164, #19738, #10994, #36391, #30725, #34302, #16696, #33564, #16882, #8346, #31276, #25216, #34113, #28244, #2274, #7601, #19547, #2091, #13471, #13851, #14031, #25582, #36580, #37135, #16321, #27868, #19917, #36767, #5303, #11180, #30906, #31095, #28418, #16509, #1901, #31457, #22753, #28056, #19176, #10621, #22200, #7788, #13284, #5480, #17063, #24839, #19366, #13666, #10810, #25398, #36948, #6427, #26136, #28602, #9274, #3015, #14584, #14216, #8893, #26508, #22940, #34666, #2639, #20094, #14398, #11368, #32386, #2826, #539, #170, #11737, #5668, #6237, #25766, #5858, #23307, #31640, #23678, #23488, #12105, #17248, #34853, #20283, #20471, #32010, #6041, #34485, #11921, #357, #29352, #17627, #37318, #8528, #29157, #11548, #25955, #3199, #37497, #31823, #14776, #28789, #26320, #35039, #20846, #9086, #35225, #23122, #8711, #17436, #28974, #20655, #32202, #17812, #3392, #14961, #24056, #33332, #4145, #6613, #30303, #3953, #6800, #36162, #1484, #725, #18001, #18761, #4328, #21224, #12297, #21036, #27083, #21410, #18375, #23871 ) ),
 .UNSPECIFIED., .F., .F., .F. ) 
 B_SPLINE_SURFACE_WITH_KNOTS ( ( 2, 2 ),
 ( 3, 2, 2, 2, 2, 2, 2, 2, 2, 2, 2, 2, 2, 2, 2, 2, 2, 2, 2, 2, 2, 2, 2, 2, 2, 2, 2, 2, 2, 2, 2, 2, 2, 2, 2, 2, 2, 2, 2, 2, 2, 2, 2, 2, 2, 2, 2, 2, 2, 2, 2, 2, 2, 2, 2, 2, 2, 2, 2, 2, 2, 2, 2, 2, 2, 2, 2, 3 ),
 ( 0.000000000000000000, 1.000000000000000000 ),
 ( 0.000000000000000000, 0.01388888888888888812, 0.02777777777777777624, 0.04166666666666666435, 0.05555555555555555247, 0.06944444444444444753, 0.08333333333333332871, 0.09722222222222222376, 0.1111111111111111049, 0.1250000000000000000, 0.1388888888888888951, 0.1527777777777777901, 0.1666666666666666574, 0.1805555555555555525, 0.1944444444444444475, 0.2083333333333333426, 0.2222222222222222099, 0.2361111111111111049, 0.2500000000000000000, 0.2638888888888888951, 0.2777777777777777901, 0.2916666666666666852, 0.3055555555555555802, 0.3194444444444444198, 0.3333333333333333148, 0.3472222222222222099, 0.3611111111111111049, 0.3750000000000000000, 0.3888888888888888951, 0.4027777777777777901, 0.4166666666666666852, 0.4305555555555555802, 0.4444444444444444198, 0.4583333333333333148, 0.4722222222222222099, 0.4861111111111111049, 0.5000000000000000000, 0.5138888888888888395, 0.5277777777777777901, 0.5416666666666666297, 0.5555555555555555802, 0.5694444444444444198, 0.5833333333333333703, 0.5972222222222222099, 0.6111111111111111605, 0.6250000000000000000, 0.6388888888888888395, 0.6527777777777777901, 0.6666666666666666297, 0.6805555555555555802, 0.6944444444444444198, 0.7083333333333333703, 0.7222222222222222099, 0.7361111111111111605, 0.7500000000000000000, 0.7638888888888888395, 0.7777777777777777901, 0.7916666666666666297, 0.8055555555555555802, 0.8194444444444444198, 0.8333333333333333703, 0.8472222222222222099, 0.8611111111111111605, 0.8750000000000000000, 0.8888888888888888395, 0.9027777777777777901, 0.9166666666666666297, 0.9258785558287927486 ),
 .UNSPECIFIED. ) 
 GEOMETRIC_REPRESENTATION_ITEM ( )  RATIONAL_B_SPLINE_SURFACE ( (
 ( 1.000000000000000000, 0.8660254037844387076, 1.000000000000000000, 0.8660254037844387076, 1.000000000000000000, 0.8660254037844387076, 1.000000000000000000, 0.8660254037844387076, 1.000000000000000000, 0.8660254037844387076, 1.000000000000000000, 0.8660254037844387076, 1.000000000000000000, 0.8660254037844387076, 1.000000000000000000, 0.8660254037844387076, 1.000000000000000000, 0.8660254037844387076, 1.000000000000000000, 0.8660254037844387076, 1.000000000000000000, 0.8660254037844387076, 1.000000000000000000, 0.8660254037844387076, 1.000000000000000000, 0.8660254037844387076, 1.000000000000000000, 0.8660254037844387076, 1.000000000000000000, 0.8660254037844387076, 1.000000000000000000, 0.8660254037844387076, 1.000000000000000000, 0.8660254037844387076, 1.000000000000000000, 0.8660254037844387076, 1.000000000000000000, 0.8660254037844387076, 1.000000000000000000, 0.8660254037844387076, 1.000000000000000000, 0.8660254037844387076, 1.000000000000000000, 0.8660254037844387076, 1.000000000000000000, 0.8660254037844387076, 1.000000000000000000, 0.8660254037844387076, 1.000000000000000000, 0.8660254037844387076, 1.000000000000000000, 0.8660254037844387076, 1.000000000000000000, 0.8660254037844387076, 1.000000000000000000, 0.8660254037844387076, 1.000000000000000000, 0.8660254037844387076, 1.000000000000000000, 0.8660254037844387076, 1.000000000000000000, 0.8660254037844387076, 1.000000000000000000, 0.8660254037844387076, 1.000000000000000000, 0.8660254037844387076, 1.000000000000000000, 0.8660254037844387076, 1.000000000000000000, 0.8660254037844387076, 1.000000000000000000, 0.8660254037844387076, 1.000000000000000000, 0.8660254037844387076, 1.000000000000000000, 0.8660254037844387076, 1.000000000000000000, 0.8660254037844387076, 1.000000000000000000, 0.8660254037844387076, 1.000000000000000000, 0.8660254037844387076, 1.000000000000000000, 0.8660254037844387076, 1.000000000000000000, 0.8660254037844387076, 1.000000000000000000, 0.8660254037844387076, 1.000000000000000000, 0.8660254037844387076, 1.000000000000000000, 0.8660254037844387076, 1.000000000000000000, 0.8660254037844387076, 1.000000000000000000, 0.8660254037844387076, 1.000000000000000000, 0.8660254037844387076, 1.000000000000000000, 0.8660254037844387076, 1.000000000000000000, 0.8660254037844387076, 1.000000000000000000, 0.8660254037844387076, 1.000000000000000000, 0.8660254037844387076, 1.000000000000000000, 0.8660254037844387076, 1.000000000000000000, 0.8660254037844387076, 1.000000000000000000, 0.8660254037844387076, 1.000000000000000000, 0.8660254037844387076, 1.000000000000000000, 0.8660254037844387076, 1.000000000000000000, 0.8660254037844387076, 1.000000000000000000, 0.8660254037844387076, 1.000000000000000000, 0.8660254037844387076, 1.000000000000000000, 0.8660254037844387076, 1.000000000000000000, 0.8660254037844387076, 1.000000000000000000, 0.8660254037844387076, 1.000000000000000000, 0.8660254037844387076, 1.000000000000000000, 0.8660254037844387076, 1.000000000000000000, 0.9111405425767590271, 0.9401542252352144136),
 ( 1.000000000000000000, 0.8660254037844387076, 1.000000000000000000, 0.8660254037844387076, 1.000000000000000000, 0.8660254037844387076, 1.000000000000000000, 0.8660254037844387076, 1.000000000000000000, 0.8660254037844387076, 1.000000000000000000, 0.8660254037844387076, 1.000000000000000000, 0.8660254037844387076, 1.000000000000000000, 0.8660254037844387076, 1.000000000000000000, 0.8660254037844387076, 1.000000000000000000, 0.8660254037844387076, 1.000000000000000000, 0.8660254037844387076, 1.000000000000000000, 0.8660254037844387076, 1.000000000000000000, 0.8660254037844387076, 1.000000000000000000, 0.8660254037844387076, 1.000000000000000000, 0.8660254037844387076, 1.000000000000000000, 0.8660254037844387076, 1.000000000000000000, 0.8660254037844387076, 1.000000000000000000, 0.8660254037844387076, 1.000000000000000000, 0.8660254037844387076, 1.000000000000000000, 0.8660254037844387076, 1.000000000000000000, 0.8660254037844387076, 1.000000000000000000, 0.8660254037844387076, 1.000000000000000000, 0.8660254037844387076, 1.000000000000000000, 0.8660254037844387076, 1.000000000000000000, 0.8660254037844387076, 1.000000000000000000, 0.8660254037844387076, 1.000000000000000000, 0.8660254037844387076, 1.000000000000000000, 0.8660254037844387076, 1.000000000000000000, 0.8660254037844387076, 1.000000000000000000, 0.8660254037844387076, 1.000000000000000000, 0.8660254037844387076, 1.000000000000000000, 0.8660254037844387076, 1.000000000000000000, 0.8660254037844387076, 1.000000000000000000, 0.8660254037844387076, 1.000000000000000000, 0.8660254037844387076, 1.000000000000000000, 0.8660254037844387076, 1.000000000000000000, 0.8660254037844387076, 1.000000000000000000, 0.8660254037844387076, 1.000000000000000000, 0.8660254037844387076, 1.000000000000000000, 0.8660254037844387076, 1.000000000000000000, 0.8660254037844387076, 1.000000000000000000, 0.8660254037844387076, 1.000000000000000000, 0.8660254037844387076, 1.000000000000000000, 0.8660254037844387076, 1.000000000000000000, 0.8660254037844387076, 1.000000000000000000, 0.8660254037844387076, 1.000000000000000000, 0.8660254037844387076, 1.000000000000000000, 0.8660254037844387076, 1.000000000000000000, 0.8660254037844387076, 1.000000000000000000, 0.8660254037844387076, 1.000000000000000000, 0.8660254037844387076, 1.000000000000000000, 0.8660254037844387076, 1.000000000000000000, 0.8660254037844387076, 1.000000000000000000, 0.8660254037844387076, 1.000000000000000000, 0.8660254037844387076, 1.000000000000000000, 0.8660254037844387076, 1.000000000000000000, 0.8660254037844387076, 1.000000000000000000, 0.8660254037844387076, 1.000000000000000000, 0.8660254037844387076, 1.000000000000000000, 0.8660254037844387076, 1.000000000000000000, 0.8660254037844387076, 1.000000000000000000, 0.8660254037844387076, 1.000000000000000000, 0.8660254037844387076, 1.000000000000000000, 0.8660254037844387076, 1.000000000000000000, 0.8660254037844387076, 1.000000000000000000, 0.8660254037844387076, 1.000000000000000000, 0.9111405425767590271, 0.9401542252352144136) ) ) 
 REPRESENTATION_ITEM ( '' )  SURFACE ( )  );
#10511=CARTESIAN_POINT ( 'NONE',  ( -13.50000000000000533, 197.2250000000000227, -23.38268590217984411 ) ) ;
#10519=CARTESIAN_POINT ( 'NONE',  ( 1.255007937094097924E-14, 199.1000000012290627, -27.00000000000000000 ) ) ;
#10521=CARTESIAN_POINT ( 'NONE',  ( 1.069080835302379631E-14, 195.6124999999999829, 27.00000000000000000 ) ) ;
#10603=CARTESIAN_POINT ( 'NONE',  ( 0.000000000000000000, 200.0000000000000000, -27.00000000000000355 ) ) ;
#10608=CARTESIAN_POINT ( 'NONE',  ( 13.62178482187501416, 195.9593750006145569, 23.59362340125806767 ) ) ;
#10621=CARTESIAN_POINT ( 'NONE',  ( -1.909035429704832693E-15, 198.2000000012290286, -31.17691453623979214 ) ) ;
#10632=CARTESIAN_POINT ( 'NONE',  ( 1.069080835302379631E-14, 195.2750000012290457, 27.00000000000000000 ) ) ;
#10643=CARTESIAN_POINT ( 'NONE',  ( -27.24356964374999635, 196.6906250006145456, 15.72908226750539384 ) ) ;
#10680=ORIENTED_EDGE ( 'NONE', *, *, #2732, .T. ) ;
#10682=CARTESIAN_POINT ( 'NONE',  ( 27.24356964375000700, 195.4906250006145001, 15.72908226750537075 ) ) ;
#10683=CARTESIAN_POINT ( 'NONE',  ( 13.62178482187501416, 197.7593750006145399, 23.59362340125806767 ) ) ;
#10684=DIRECTION ( 'NONE',  ( -0.000000000000000000, -1.000000000000000000, -0.000000000000000000 ) ) ;
#10700=CARTESIAN_POINT ( 'NONE',  ( -27.00000000000000355, 196.8500000000000227, 0.000000000000000000 ) ) ;
#10709=CARTESIAN_POINT ( 'NONE',  ( 0.000000000000000000, 2.000000000000000000, -5.000000000000000000 ) ) ;
#10726=CARTESIAN_POINT ( 'NONE',  ( -3.253724281355068545E-15, 195.9500000012290002, -27.00000000000000000 ) ) ;
#10806=CARTESIAN_POINT ( 'NONE',  ( 0.000000000000000000, 200.0000000000000000, 0.000000000000000000 ) ) ;
#10810=CARTESIAN_POINT ( 'NONE',  ( -27.00000000000000355, 197.8625000012290513, 0.000000000000000000 ) ) ;
#10825=CARTESIAN_POINT ( 'NONE',  ( 26.99999999999999645, 198.0125000000000739, -15.58845726811990495 ) ) ;
#10831=CARTESIAN_POINT ( 'NONE',  ( 5.778771075727756162E-15, 196.7656250006145342, 31.45816453501075927 ) ) ;
#10836=SHAPE_REPRESENTATION ( 'Cylinder', ( #17215 ), #33555 ) ;
#10865=EDGE_CURVE ( 'NONE', #1101, #17216, #6839, .T. ) ;
#10871=CARTESIAN_POINT ( 'NONE',  ( 27.24356964375000700, 195.0406250006145399, 15.72908226750537075 ) ) ;
#10872=CARTESIAN_POINT ( 'NONE',  ( -1.926257025242585782E-15, 198.8468750006145740, -31.45816453501075927 ) ) ;
#10876=CARTESIAN_POINT ( 'NONE',  ( 13.49999999999999645, 196.3625000012290513, -23.38268590217984766 ) ) ;
#10880=VERTEX_POINT ( 'NONE', #24623 ) ;
#10888=CARTESIAN_POINT ( 'NONE',  ( -27.00000000000000355, 195.9500000000000171, 0.000000000000000000 ) ) ;
#10902=FILL_AREA_STYLE_COLOUR ( '', #22059 ) ;
#10941=CARTESIAN_POINT ( 'NONE',  ( -27.00000000000000355, 196.5125000012290570, 0.000000000000000000 ) ) ;
#10944=ORIENTED_EDGE ( 'NONE', *, *, #19321, .T. ) ;
#10951=CARTESIAN_POINT ( 'NONE',  ( -13.50000000000000533, 199.4750000000000227, -23.38268590217984411 ) ) ;
#10960=DIRECTION ( 'NONE',  ( 0.000000000000000000, 0.000000000000000000, -1.000000000000000000 ) ) ;
#10967=CARTESIAN_POINT ( 'NONE',  ( 0.000000000000000000, 200.0000000000000000, -27.00000000000000355 ) ) ;
#10994=CARTESIAN_POINT ( 'NONE',  ( -13.50000000000000533, 199.5875000012290457, -23.38268590217984411 ) ) ;
#11019=CARTESIAN_POINT ( 'NONE',  ( 27.24356964374999635, 196.4656250006145228, -15.72908226750539029 ) ) ;
#11022=CYLINDRICAL_SURFACE ( 'NONE', #8359, 27.00000000000000355 ) ;
#11036=( BOUNDED_CURVE ( )  B_SPLINE_CURVE ( 2, ( #37297, #7948, #17228, #2065, #11346, #22918, #34463, #25192, #28766 ),
 .UNSPECIFIED., .F., .T. ) 
 B_SPLINE_CURVE_WITH_KNOTS ( ( 3, 2, 2, 2, 3 ),
 ( 0.4791666666666666852, 0.4861111111111111049, 0.5000000000000000000, 0.5138888888888888395, 0.5208333333333333703 ),
 .UNSPECIFIED. ) 
 CURVE ( )  GEOMETRIC_REPRESENTATION_ITEM ( )  RATIONAL_B_SPLINE_CURVE ( ( 0.9330127018922194093, 0.9330127018922196314, 1.000000000000000000, 0.8660254037844387076, 1.000000000000000000, 0.8660254037844387076, 1.000000000000000000, 0.9330127018922187432, 0.9330127018922192983 ) ) 
 REPRESENTATION_ITEM ( '' )  );
#11057=CARTESIAN_POINT ( 'NONE',  ( 27.24356964375000345, 195.0781250006145342, -3.336375036156643733E-15 ) ) ;
#11058=CARTESIAN_POINT ( 'NONE',  ( -27.24356964375000345, 198.5093750006145399, 0.000000000000000000 ) ) ;
#11059=CARTESIAN_POINT ( 'NONE',  ( 0.000000000000000000, 2.000000000000000000, 0.000000000000000000 ) ) ;
#11062=CARTESIAN_POINT ( 'NONE',  ( 27.00000000000000355, 196.2875000012290343, -3.306546357697854128E-15 ) ) ;
#11069=CARTESIAN_POINT ( 'NONE',  ( -4.694659320240884604E-14, 197.0750000012290570, 27.00000000000000000 ) ) ;
#11075=CARTESIAN_POINT ( 'NONE',  ( 13.49999999999999645, 196.2500000000000000, -23.38268590217984766 ) ) ;
#11180=CARTESIAN_POINT ( 'NONE',  ( 26.99999999999999645, 198.5750000012290286, -15.58845726811990495 ) ) ;
#11243=CARTESIAN_POINT ( 'NONE',  ( -1.926257025242585782E-15, 197.4968750006145513, -31.45816453501075927 ) ) ;
#11246=CARTESIAN_POINT ( 'NONE',  ( 1.120210788295102201E-13, 195.8375000000000057, -27.00000000000000711 ) ) ;
#11249=APPLICATION_CONTEXT ( 'automotive_design' ) ;
#11255=CARTESIAN_POINT ( 'NONE',  ( -13.50000000000000533, 195.8750000000000284, -23.38268590217984411 ) ) ;
#11257=EDGE_LOOP ( 'NONE', ( #6678, #84, #2808, #28550 ) ) ;
#11262=( BOUNDED_CURVE ( )  B_SPLINE_CURVE ( 2, ( #32450, #28852, #3077, #17128, #26196, #14277, #2886, #14838, #11428 ),
 .UNSPECIFIED., .F., .F. ) 
 B_SPLINE_CURVE_WITH_KNOTS ( ( 3, 2, 2, 2, 3 ),
 ( 0.8541666666666667407, 0.8611111111111111605, 0.8750000000000000000, 0.8888888888888888395, 0.8958333333333333703 ),
 .UNSPECIFIED. ) 
 CURVE ( )  GEOMETRIC_REPRESENTATION_ITEM ( )  RATIONAL_B_SPLINE_CURVE ( ( 0.9330127018922192983, 0.9330127018922198534, 1.000000000000000000, 0.8660254037844387076, 1.000000000000000000, 0.8660254037844387076, 1.000000000000000000, 0.9330127018922187432, 0.9330127018922192983 ) ) 
 REPRESENTATION_ITEM ( '' )  );
#11264=CARTESIAN_POINT ( 'NONE',  ( 27.00000000000000355, 196.1750000000000114, -3.306546357697854128E-15 ) ) ;
#11265=ORIENTED_EDGE ( 'NONE', *, *, #34880, .T. ) ;
#11296=ADVANCED_FACE ( 'NONE', ( #31428 ), #5449, .T. ) ;
#11319=CARTESIAN_POINT ( 'NONE',  ( 0.000000000000000000, 200.0000000000000000, 0.000000000000000000 ) ) ;
#11328=DIRECTION ( 'NONE',  ( -0.000000000000000000, -1.000000000000000000, -0.000000000000000000 ) ) ;
#11337=CYLINDRICAL_SURFACE ( 'NONE', #16283, 27.00000000000000355 ) ;
#11344=ADVANCED_FACE ( 'NONE', ( #2239 ), #11337, .T. ) ;
#11346=CARTESIAN_POINT ( 'NONE',  ( -27.00000000000000355, 197.3000000000000114, 0.000000000000000000 ) ) ;
#11360=ORIENTED_EDGE ( 'NONE', *, *, #29019, .T. ) ;
#11368=CARTESIAN_POINT ( 'NONE',  ( 26.99999999999999645, 197.2250000012290059, -15.58845726811990495 ) ) ;
#11381=CARTESIAN_POINT ( 'NONE',  ( 3.306546357697854128E-15, 0.000000000000000000, 27.00000000000000355 ) ) ;
#11396=CARTESIAN_POINT ( 'NONE',  ( 13.62178482187499640, 199.7093750006145285, -23.59362340125807123 ) ) ;
#11428=CARTESIAN_POINT ( 'NONE',  ( -1.045839947578415010E-13, 195.1625000000000512, 27.00000000000000355 ) ) ;
#11429=CARTESIAN_POINT ( 'NONE',  ( -13.62178482187498396, 195.8843750006145399, 23.59362340125808188 ) ) ;
#11448=CARTESIAN_POINT ( 'NONE',  ( -27.24356964375000345, 199.8593750006145342, 0.000000000000000000 ) ) ;
#11454=CYLINDRICAL_SURFACE ( 'NONE', #1565, 27.00000000000000355 ) ;
#11485=CARTESIAN_POINT ( 'NONE',  ( -13.50000000000000533, 197.7875000012290627, -23.38268590217984411 ) ) ;
#11501=CYLINDRICAL_SURFACE ( 'NONE', #28340, 27.00000000000000355 ) ;
#11505=( BOUNDED_CURVE ( )  B_SPLINE_CURVE ( 2, ( #30841, #37255, #22692, #5238, #1837, #37069, #13598, #2205, #5050 ),
 .UNSPECIFIED., .F., .F. ) 
 B_SPLINE_CURVE_WITH_KNOTS ( ( 3, 2, 2, 2, 3 ),
 ( 0.3541666666666666852, 0.3611111111111111049, 0.3750000000000000000, 0.3888888888888888951, 0.3958333333333333703 ),
 .UNSPECIFIED. ) 
 CURVE ( )  GEOMETRIC_REPRESENTATION_ITEM ( )  RATIONAL_B_SPLINE_CURVE ( ( 0.9330127018922194093, 0.9330127018922196314, 1.000000000000000000, 0.8660254037844387076, 1.000000000000000000, 0.8660254037844387076, 1.000000000000000000, 0.9330127018922190762, 0.9330127018922194093 ) ) 
 REPRESENTATION_ITEM ( '' )  );
#11516=VERTEX_POINT ( 'NONE', #26106 ) ;
#11548=CARTESIAN_POINT ( 'NONE',  ( -13.49999999999998401, 196.1375000012290286, 23.38268590217985476 ) ) ;
#11579=CARTESIAN_POINT ( 'NONE',  ( -27.24356964374999279, 199.4468750006145399, 15.72908226750539384 ) ) ;
#11587=ORIENTED_EDGE ( 'NONE', *, *, #16417, .F. ) ;
#11589=CARTESIAN_POINT ( 'NONE',  ( -27.24356964374999635, 198.9406250006145171, 15.72908226750539384 ) ) ;
#11610=CARTESIAN_POINT ( 'NONE',  ( 5.778771075727756162E-15, 195.9218750006145342, 31.45816453501075927 ) ) ;
#11620=CARTESIAN_POINT ( 'NONE',  ( -3.253724281355068545E-15, 197.3000000012290229, -27.00000000000000000 ) ) ;
#11628=CARTESIAN_POINT ( 'NONE',  ( 13.50000000000001421, 195.6500000000000057, 23.38268590217984055 ) ) ;
#11649=DIRECTION ( 'NONE',  ( -0.000000000000000000, -1.000000000000000000, -0.000000000000000000 ) ) ;
#11655=CARTESIAN_POINT ( 'NONE',  ( 13.62178482187501416, 199.0531250006145285, 23.59362340125806767 ) ) ;
#11671=CARTESIAN_POINT ( 'NONE',  ( 13.49999999999999645, 197.5999999999999943, -23.38268590217984766 ) ) ;
#11675=CARTESIAN_POINT ( 'NONE',  ( 1.120210788295102201E-13, 196.4000000012290741, -27.00000000000000711 ) ) ;
#11680=ORIENTED_EDGE ( 'NONE', *, *, #15193, .T. ) ;
#11683=CARTESIAN_POINT ( 'NONE',  ( 0.000000000000000000, 200.0000000000000000, -27.00000000000000355 ) ) ;
#11711=CARTESIAN_POINT ( 'NONE',  ( 1.069080835302379631E-14, 199.6625000000000227, 27.00000000000000000 ) ) ;
#11712=DIRECTION ( 'NONE',  ( -0.000000000000000000, -1.000000000000000000, -0.000000000000000000 ) ) ;
#11737=CARTESIAN_POINT ( 'NONE',  ( -13.49999999999998401, 197.0375000012290627, 23.38268590217985476 ) ) ;
#11748=CARTESIAN_POINT ( 'NONE',  ( 0.000000000000000000, 2.000000000000000000, 0.000000000000000000 ) ) ;
#11756=ORIENTED_EDGE ( 'NONE', *, *, #15622, .T. ) ;
#11779=CARTESIAN_POINT ( 'NONE',  ( -1.926257025242585782E-15, 197.8906250006145342, -31.45816453501075927 ) ) ;
#11792=ADVANCED_FACE ( 'NONE', ( #18342 ), #4483, .F. ) ;
#11799=CARTESIAN_POINT ( 'NONE',  ( 5.778771075727756162E-15, 195.0218750006145569, 31.45816453501075927 ) ) ;
#11815=CARTESIAN_POINT ( 'NONE',  ( -27.24356964374999990, 197.5718750006145399, -15.72908226750537786 ) ) ;
#11821=CARTESIAN_POINT ( 'NONE',  ( -27.00000000000000355, 195.4625000000000057, -15.58845726811989429 ) ) ;
#11851=CARTESIAN_POINT ( 'NONE',  ( 1.069080835302379631E-14, 197.9750000012290343, 27.00000000000000000 ) ) ;
#11861=CARTESIAN_POINT ( 'NONE',  ( -1.909035429704832693E-15, 198.9875000000000114, -31.17691453623979214 ) ) ;
#11874=FACE_OUTER_BOUND ( 'NONE', #25613, .T. ) ;
#11921=CARTESIAN_POINT ( 'NONE',  ( -1.909035429704832693E-15, 196.4000000012290457, -31.17691453623979214 ) ) ;
#11933=AXIS2_PLACEMENT_3D ( 'NONE', #10806, #2270, #2455 ) ;
#11942=CARTESIAN_POINT ( 'NONE',  ( -27.24356964374999990, 196.6718750006145342, -15.72908226750537786 ) ) ;
#11954=CARTESIAN_POINT ( 'NONE',  ( -27.24356964375000345, 199.4093750006145456, 0.000000000000000000 ) ) ;
#11964=CARTESIAN_POINT ( 'NONE',  ( 27.24356964375000345, 198.2281250006145399, -3.336375036156643733E-15 ) ) ;
#11967=AXIS2_PLACEMENT_3D ( 'NONE', #199, #23332, #2668 ) ;
#11986=CARTESIAN_POINT ( 'NONE',  ( 13.62178482187499640, 197.0093750006145399, -23.59362340125807123 ) ) ;
#11987=CARTESIAN_POINT ( 'NONE',  ( 7.234628195640337545, 198.1799038117967200, -26.99999999999999289 ) ) ;
#12003=CARTESIAN_POINT ( 'NONE',  ( 13.62178482187499640, 197.9093750006145456, -23.59362340125807123 ) ) ;
#12041=ORIENTED_EDGE ( 'NONE', *, *, #34859, .T. ) ;
#12043=CARTESIAN_POINT ( 'NONE',  ( 0.000000000000000000, 200.0000000000000000, -27.00000000000000355 ) ) ;
#12048=CARTESIAN_POINT ( 'NONE',  ( -27.00000000000000355, 199.5124999999999886, -15.58845726811989429 ) ) ;
#12091=CARTESIAN_POINT ( 'NONE',  ( 27.00000000000000355, 196.6250000000000284, -3.306546357697854128E-15 ) ) ;
#12103=AXIS2_PLACEMENT_3D ( 'NONE', #36595, #1915, #19002 ) ;
#12105=CARTESIAN_POINT ( 'NONE',  ( 27.00000000000001066, 196.7000000012290286, 15.58845726811988897 ) ) ;
#12123=CARTESIAN_POINT ( 'NONE',  ( 27.00000000000001421, 194.9000000012290457, 15.58845726811988897 ) ) ;
#12125=CARTESIAN_POINT ( 'NONE',  ( -13.62178482187500528, 195.7343750006145626, -23.59362340125807123 ) ) ;
#12137=CARTESIAN_POINT ( 'NONE',  ( -13.62178482187500528, 198.8843750006145399, -23.59362340125807123 ) ) ;
#12148=FACE_OUTER_BOUND ( 'NONE', #18874, .T. ) ;
#12173=CARTESIAN_POINT ( 'NONE',  ( -27.24356964375000345, 194.9093750006145456, 0.000000000000000000 ) ) ;
#12174=DIRECTION ( 'NONE',  ( -0.000000000000000000, -1.000000000000000000, -0.000000000000000000 ) ) ;
#12190=CARTESIAN_POINT ( 'NONE',  ( -1.926257025242585782E-15, 197.4968750006145513, -31.45816453501075927 ) ) ;
#12219=CARTESIAN_POINT ( 'NONE',  ( 27.24356964374999279, 199.1656250006145399, -15.72908226750539207 ) ) ;
#12236=CARTESIAN_POINT ( 'NONE',  ( 27.00000000000001066, 199.7375000000000114, 15.58845726811988897 ) ) ;
#12243=CARTESIAN_POINT ( 'NONE',  ( 5.438367727407757144E-14, 198.2000000012290002, -27.00000000000000000 ) ) ;
#12297=CARTESIAN_POINT ( 'NONE',  ( 5.727106289114498080E-15, 194.8250000012290570, 31.17691453623979214 ) ) ;
#12304=CARTESIAN_POINT ( 'NONE',  ( -1.045839947578415010E-13, 196.0625000000000284, 27.00000000000000355 ) ) ;
#12314=CARTESIAN_POINT ( 'NONE',  ( -27.00000000000000355, 199.0999999999999943, 0.000000000000000000 ) ) ;
#12318=AXIS2_PLACEMENT_3D ( 'NONE', #35104, #12174, #32453 ) ;
#12319=CARTESIAN_POINT ( 'NONE',  ( -1.926257025242585782E-15, 196.1468750006145285, -31.45816453501075927 ) ) ;
#12327=CARTESIAN_POINT ( 'NONE',  ( 13.49999999999999645, 198.5000000000000000, -23.38268590217984766 ) ) ;
#12329=CARTESIAN_POINT ( 'NONE',  ( -1.926257025242585782E-15, 197.9468750006145399, -31.45816453501076637 ) ) ;
#12338=CARTESIAN_POINT ( 'NONE',  ( 0.000000000000000000, 2.000000000000000000, 0.000000000000000000 ) ) ;
#12342=CARTESIAN_POINT ( 'NONE',  ( 27.24356964374999635, 197.3656250006145285, -15.72908226750539029 ) ) ;
#12349=CARTESIAN_POINT ( 'NONE',  ( 26.99999999999999645, 197.1125000000000114, -15.58845726811990495 ) ) ;
#12350=EDGE_CURVE ( 'NONE', #26752, #55, #3495, .T. ) ;
#12368=CARTESIAN_POINT ( 'NONE',  ( -13.62178482187498396, 197.6281250006145171, 23.59362340125808188 ) ) ;
#12383=CARTESIAN_POINT ( 'NONE',  ( -27.24356964374999635, 198.0968750006145456, 15.72908226750539384 ) ) ;
#12408=CARTESIAN_POINT ( 'NONE',  ( 5.778771075727756162E-15, 198.5656250006145456, 31.45816453501076637 ) ) ;
#12410=CARTESIAN_POINT ( 'NONE',  ( -27.12178482187499995, 199.9296875003072671, 0.000000000000000000 ) ) ;
#12428=CARTESIAN_POINT ( 'NONE',  ( 27.00000000000000355, 199.3249999999999886, -3.306546357697854128E-15 ) ) ;
#12444=DIRECTION ( 'NONE',  ( 0.000000000000000000, -1.000000000000000000, 0.000000000000000000 ) ) ;
#12493=EDGE_CURVE ( 'NONE', #1851, #2775, #14429, .T. ) ;
#12511=CARTESIAN_POINT ( 'NONE',  ( 1.255007937094097924E-14, 199.1000000012290627, -27.00000000000000000 ) ) ;
#12513=CARTESIAN_POINT ( 'NONE',  ( -1.926257025242585782E-15, 195.2468750006145513, -31.45816453501075927 ) ) ;
#12515=EDGE_LOOP ( 'NONE', ( #3784, #21961, #25481, #8100 ) ) ;
#12522=CARTESIAN_POINT ( 'NONE',  ( -4.694659320240884604E-14, 197.5250000012290172, 27.00000000000000000 ) ) ;
#12523=CARTESIAN_POINT ( 'NONE',  ( -3.253724281355068545E-15, 198.9874999999999829, -27.00000000000000000 ) ) ;
#12525=CARTESIAN_POINT ( 'NONE',  ( 13.62178482187499640, 196.5593750006145513, -23.59362340125807123 ) ) ;
#12538=CARTESIAN_POINT ( 'NONE',  ( 5.778771075727756162E-15, 195.8656250006145285, 31.45816453501075927 ) ) ;
#12561=CARTESIAN_POINT ( 'NONE',  ( 27.24356964374999635, 197.3656250006145285, -15.72908226750539029 ) ) ;
#12600=CARTESIAN_POINT ( 'NONE',  ( 27.24356964375000700, 196.3906250006145342, 15.72908226750537075 ) ) ;
#12615=CARTESIAN_POINT ( 'NONE',  ( -27.00000000000000355, 200.0000000000000000, 0.000000000000000000 ) ) ;
#12685=CARTESIAN_POINT ( 'NONE',  ( 7.234628195640269155, 196.0825961894323939, 27.00000000000003197 ) ) ;
#12706=CARTESIAN_POINT ( 'NONE',  ( 27.24356964375000345, 196.4843750006145626, -3.336375036156643733E-15 ) ) ;
#12717=CARTESIAN_POINT ( 'NONE',  ( -27.00000000000000355, 199.6250000012290400, -15.58845726811989429 ) ) ;
#12721=CARTESIAN_POINT ( 'NONE',  ( 13.62178482187499640, 196.5031250006145456, -23.59362340125807123 ) ) ;
#12734=ORIENTED_EDGE ( 'NONE', *, *, #19321, .F. ) ;
#12748=CARTESIAN_POINT ( 'NONE',  ( 27.24356964375000345, 199.1281250006145171, -3.336375036156643733E-15 ) ) ;
#12764=CARTESIAN_POINT ( 'NONE',  ( 3.061616997868383043E-15, 200.0000000000000000, 25.00000000000000000 ) ) ;
#12769=DIRECTION ( 'NONE',  ( 0.000000000000000000, -0.000000000000000000, 1.000000000000000000 ) ) ;
#12785=CARTESIAN_POINT ( 'NONE',  ( 13.62178482187501416, 198.6031250006145399, 23.59362340125806767 ) ) ;
#12799=CARTESIAN_POINT ( 'NONE',  ( -13.50000000000000533, 198.1250000000000284, -23.38268590217984411 ) ) ;
#12806=CARTESIAN_POINT ( 'NONE',  ( -26.99999999999999645, 199.2500000012290116, 15.58845726811991561 ) ) ;
#12815=CARTESIAN_POINT ( 'NONE',  ( 0.000000000000000000, 200.0000000000000000, 0.000000000000000000 ) ) ;
#12827=CARTESIAN_POINT ( 'NONE',  ( -7.234628195640354420, 196.1549038117966859, 26.99999999999996803 ) ) ;
#12862=EDGE_CURVE ( 'NONE', #5775, #5529, #3691, .T. ) ;
#12890=EDGE_CURVE ( 'NONE', #36429, #8730, #4066, .T. ) ;
#12898=CARTESIAN_POINT ( 'NONE',  ( 27.24356964375000345, 198.2843750006145456, -3.336375036156643733E-15 ) ) ;
#12912=CARTESIAN_POINT ( 'NONE',  ( -27.24356964374999990, 196.6156250006145285, -15.72908226750537786 ) ) ;
#12924=CARTESIAN_POINT ( 'NONE',  ( 0.000000000000000000, 200.0000000000000000, 0.000000000000000000 ) ) ;
#12938=CARTESIAN_POINT ( 'NONE',  ( -1.926257025242585782E-15, 198.3406250006145228, -31.45816453501075927 ) ) ;
#12964=ADVANCED_FACE ( 'NONE', ( #29655 ), #30310, .F. ) ;
#12979=CARTESIAN_POINT ( 'NONE',  ( -13.62178482187500528, 197.0281250006145228, -23.59362340125807123 ) ) ;
#12988=AXIS2_PLACEMENT_3D ( 'NONE', #17736, #3316, #14887 ) ;
#12996=CARTESIAN_POINT ( 'NONE',  ( 13.50000000000001421, 197.9000000000000341, 23.38268590217984055 ) ) ;
#13003=CARTESIAN_POINT ( 'NONE',  ( 1.069080835302379631E-14, 199.3250000012290286, 27.00000000000000000 ) ) ;
#13017=CARTESIAN_POINT ( 'NONE',  ( 6.123233995736766282E-16, 2.000000000000000000, 5.000000000000000000 ) ) ;
#13054=EDGE_CURVE ( 'NONE', #15189, #21803, #28478, .T. ) ;
#13067=CARTESIAN_POINT ( 'NONE',  ( 26.99999999999999645, 196.2125000000000057, -15.58845726811990495 ) ) ;
#13072=DIRECTION ( 'NONE',  ( -0.000000000000000000, -1.000000000000000000, -0.000000000000000000 ) ) ;
#13087=CARTESIAN_POINT ( 'NONE',  ( 13.62178482187501416, 197.3093750006145513, 23.59362340125806767 ) ) ;
#13098=CARTESIAN_POINT ( 'NONE',  ( 27.24356964375000345, 197.3281250006145342, -3.336375036156643733E-15 ) ) ;
#13124=CARTESIAN_POINT ( 'NONE',  ( -27.24356964374999635, 198.4906250006145569, 15.72908226750539384 ) ) ;
#13142=EDGE_CURVE ( 'NONE', #2631, #36062, #8376, .T. ) ;
#13161=CARTESIAN_POINT ( 'NONE',  ( 13.62178482187499640, 196.5031250006145456, -23.59362340125807123 ) ) ;
#13179=CARTESIAN_POINT ( 'NONE',  ( -1.909035429704832693E-15, 198.5374999999999943, -31.17691453623979214 ) ) ;
#13180=VERTEX_POINT ( 'NONE', #23897 ) ;
#13182=ORIENTED_EDGE ( 'NONE', *, *, #24015, .T. ) ;
#13187=CARTESIAN_POINT ( 'NONE',  ( -7.234628195640316228, 196.3075961894323598, -27.00000000000000000 ) ) ;
#13259=CARTESIAN_POINT ( 'NONE',  ( -13.50000000000000533, 195.5375000012290343, -23.38268590217984411 ) ) ;
#13269=DIRECTION ( 'NONE',  ( -0.000000000000000000, -1.000000000000000000, -0.000000000000000000 ) ) ;
#13273=CARTESIAN_POINT ( 'NONE',  ( -27.24356964375000345, 195.3218750006145399, -15.72908226750537786 ) ) ;
#13284=CARTESIAN_POINT ( 'NONE',  ( 27.00000000000000355, 198.0875000012290457, -3.306546357697854128E-15 ) ) ;
#13303=ORIENTED_EDGE ( 'NONE', *, *, #8939, .T. ) ;
#13307=CARTESIAN_POINT ( 'NONE',  ( 27.24356964375000700, 196.8406250006145513, 15.72908226750537075 ) ) ;
#13348=CARTESIAN_POINT ( 'NONE',  ( 5.778771075727756162E-15, 198.6218750006145513, 31.45816453501075927 ) ) ;
#13363=CARTESIAN_POINT ( 'NONE',  ( -1.909035429704832693E-15, 197.1875000000000284, -31.17691453623979214 ) ) ;
#13394=( BOUNDED_CURVE ( )  B_SPLINE_CURVE ( 2, ( #30862, #33889, #13810, #25539, #33515, #16093, #10951, #28011, #2044 ),
 .UNSPECIFIED., .F., .F. ) 
 B_SPLINE_CURVE_WITH_KNOTS ( ( 3, 2, 2, 2, 3 ),
 ( 0.06250000000000000000, 0.06944444444444444753, 0.08333333333333332871, 0.09722222222222222376, 0.1041666666666666713 ),
 .UNSPECIFIED. ) 
 CURVE ( )  GEOMETRIC_REPRESENTATION_ITEM ( )  RATIONAL_B_SPLINE_CURVE ( ( 0.9330127018922194093, 0.9330127018922194093, 1.000000000000000000, 0.8660254037844387076, 1.000000000000000000, 0.8660254037844387076, 1.000000000000000000, 0.9330127018922192983, 0.9330127018922194093 ) ) 
 REPRESENTATION_ITEM ( '' )  );
#13460=CARTESIAN_POINT ( 'NONE',  ( -27.24356964375000345, 194.9093750006145456, 0.000000000000000000 ) ) ;
#13471=CARTESIAN_POINT ( 'NONE',  ( 27.00000000000000355, 198.9875000012290229, -3.306546357697854128E-15 ) ) ;
#13483=CARTESIAN_POINT ( 'NONE',  ( 27.00000000000000355, 199.3249999999999886, -3.306546357697854128E-15 ) ) ;
#13491=CARTESIAN_POINT ( 'NONE',  ( -27.24356964374999990, 197.0656250006145171, -15.72908226750537786 ) ) ;
#13523=( GEOMETRIC_REPRESENTATION_CONTEXT ( 3 ) GLOBAL_UNCERTAINTY_ASSIGNED_CONTEXT ( ( #27908 ) ) GLOBAL_UNIT_ASSIGNED_CONTEXT ( ( #34024, #30449, #8618 ) ) REPRESENTATION_CONTEXT ( 'NONE', 'WORKASPACE' ) );
#13530=CARTESIAN_POINT ( 'NONE',  ( -26.99999999999999645, 197.4500000012290002, 15.58845726811991561 ) ) ;
#13533=CARTESIAN_POINT ( 'NONE',  ( 13.62178482187499640, 195.6031250006145115, -23.59362340125807123 ) ) ;
#13534=CARTESIAN_POINT ( 'NONE',  ( 13.62178482187501416, 198.6593750006145456, 23.59362340125806767 ) ) ;
#13535=CARTESIAN_POINT ( 'NONE',  ( 0.000000000000000000, 200.0000000000000000, 0.000000000000000000 ) ) ;
#13537=DIRECTION ( 'NONE',  ( 0.000000000000000000, -1.000000000000000000, 0.000000000000000000 ) ) ;
#13551=CARTESIAN_POINT ( 'NONE',  ( -1.909035429704832693E-15, 196.7374999999999829, -31.17691453623979214 ) ) ;
#13598=CARTESIAN_POINT ( 'NONE',  ( 13.50000000000001421, 197.5625000012290400, 23.38268590217984055 ) ) ;
#13647=DIRECTION ( 'NONE',  ( 0.000000000000000000, 1.000000000000000000, 0.000000000000000000 ) ) ;
#13653=ORIENTED_EDGE ( 'NONE', *, *, #33199, .T. ) ;
#13666=CARTESIAN_POINT ( 'NONE',  ( -26.99999999999998934, 197.9000000012290172, 15.58845726811991561 ) ) ;
#13680=CARTESIAN_POINT ( 'NONE',  ( 1.069080835302379631E-14, 195.2750000012290457, 27.00000000000000000 ) ) ;
#13683=CARTESIAN_POINT ( 'NONE',  ( -4.694659320240884604E-14, 197.8625000000000114, 27.00000000000000000 ) ) ;
#13689=CARTESIAN_POINT ( 'NONE',  ( -27.24356964374999990, 196.6156250006145285, -15.72908226750537786 ) ) ;
#13692=CARTESIAN_POINT ( 'NONE',  ( 5.438367727407757775E-14, 198.2000000012290002, -27.00000000000000355 ) ) ;
#13729=CARTESIAN_POINT ( 'NONE',  ( -13.62178482187498396, 194.9281250006145569, 23.59362340125808188 ) ) ;
#13730=CARTESIAN_POINT ( 'NONE',  ( 13.62178482187499640, 199.2593750006145399, -23.59362340125807123 ) ) ;
#13747=CARTESIAN_POINT ( 'NONE',  ( 27.00000000000001066, 195.2375000000000114, 15.58845726811988897 ) ) ;
#13800=ORIENTED_EDGE ( 'NONE', *, *, #33199, .F. ) ;
#13807=CIRCLE ( 'NONE', #11967, 5.000000000000000000 ) ;
#13810=CARTESIAN_POINT ( 'NONE',  ( -13.49999999999998401, 199.6250000000000284, 23.38268590217985476 ) ) ;
#13851=CARTESIAN_POINT ( 'NONE',  ( 27.00000000000001066, 198.9500000012290570, 15.58845726811988897 ) ) ;
#13865=CARTESIAN_POINT ( 'NONE',  ( 7.234628195640337545, 198.0674038105676971, -26.99999999999999289 ) ) ;
#13872=CARTESIAN_POINT ( 'NONE',  ( 3.306546357697854128E-15, 200.0000000000000000, 27.00000000000000355 ) ) ;
#13873=EDGE_CURVE ( 'NONE', #16548, #25843, #22344, .T. ) ;
#13874=CARTESIAN_POINT ( 'NONE',  ( -13.62178482187498396, 196.7281250006145399, 23.59362340125808188 ) ) ;
#13900=DIRECTION ( 'NONE',  ( 1.000000000000000000, 0.000000000000000000, -0.000000000000000000 ) ) ;
#13911=CARTESIAN_POINT ( 'NONE',  ( -13.62178482187498396, 196.2781250006145228, 23.59362340125808188 ) ) ;
#13912=CARTESIAN_POINT ( 'NONE',  ( -27.24356964374999635, 198.5468750006145626, 15.72908226750539384 ) ) ;
#13915=CARTESIAN_POINT ( 'NONE',  ( 13.49999999999999645, 195.8000000000000114, -23.38268590217984766 ) ) ;
#13929=CARTESIAN_POINT ( 'NONE',  ( -13.50000000000000533, 195.8750000000000284, -23.38268590217984411 ) ) ;
#13982=CARTESIAN_POINT ( 'NONE',  ( -3.253724281355068545E-15, 195.9500000012290002, -27.00000000000000355 ) ) ;
#14020=EDGE_CURVE ( 'NONE', #36971, #34798, #4183, .T. ) ;
#14031=CARTESIAN_POINT ( 'NONE',  ( 13.50000000000001421, 198.9125000012290343, 23.38268590217984055 ) ) ;
#14055=AXIS2_PLACEMENT_3D ( 'NONE', #34089, #37109, #8139 ) ;
#14059=DIRECTION ( 'NONE',  ( 0.000000000000000000, 0.000000000000000000, -1.000000000000000000 ) ) ;
#14089=CARTESIAN_POINT ( 'NONE',  ( 13.49999999999999645, 195.0125000012290570, -23.38268590217984766 ) ) ;
#14092=CARTESIAN_POINT ( 'NONE',  ( -27.24356964375000345, 196.2031250006145342, 0.000000000000000000 ) ) ;
#14093=CARTESIAN_POINT ( 'NONE',  ( -13.62178482187498396, 198.5843750006145569, 23.59362340125808188 ) ) ;
#14096=CARTESIAN_POINT ( 'NONE',  ( 7.234628195640363302, 195.8174038105676402, -26.99999999999996803 ) ) ;
#14110=CARTESIAN_POINT ( 'NONE',  ( -27.00000000000000355, 195.9125000000000796, -15.58845726811989429 ) ) ;
#14185=DIRECTION ( 'NONE',  ( 0.000000000000000000, 0.000000000000000000, -1.000000000000000000 ) ) ;
#14216=CARTESIAN_POINT ( 'NONE',  ( 5.727106289114498080E-15, 197.5250000012290457, 31.17691453623979214 ) ) ;
#14247=CARTESIAN_POINT ( 'NONE',  ( 5.778771075727756162E-15, 198.6218750006145513, 31.45816453501076637 ) ) ;
#14277=CARTESIAN_POINT ( 'NONE',  ( 27.00000000000001421, 195.2375000000000114, 15.58845726811988897 ) ) ;
#14278=CARTESIAN_POINT ( 'NONE',  ( -27.24356964374999990, 195.3218750006145399, -15.72908226750537786 ) ) ;
#14281=CARTESIAN_POINT ( 'NONE',  ( -20.68320042480036491, 194.9994763866750134, -17.35526491262920246 ) ) ;
#14287=ORIENTED_EDGE ( 'NONE', *, *, #37043, .F. ) ;
#14297=CARTESIAN_POINT ( 'NONE',  ( 13.62178482187499640, 199.2593750006145399, -23.59362340125807123 ) ) ;
#14316=CARTESIAN_POINT ( 'NONE',  ( -27.12178482187499995, 199.7328125009217956, 0.000000000000000000 ) ) ;
#14319=ORIENTED_EDGE ( 'NONE', *, *, #33589, .F. ) ;
#14377=CARTESIAN_POINT ( 'NONE',  ( 7.234628195640309123, 198.6299038117966802, -27.00000000000000711 ) ) ;
#14398=CARTESIAN_POINT ( 'NONE',  ( 13.49999999999999645, 197.2625000012290286, -23.38268590217984766 ) ) ;
#14428=CARTESIAN_POINT ( 'NONE',  ( -13.62178482187500528, 198.4343750006145228, -23.59362340125807123 ) ) ;
#14429=CIRCLE ( 'NONE', #35606, 27.00000000000000355 ) ;
#14439=CARTESIAN_POINT ( 'NONE',  ( 27.24356964375000345, 199.5781250006145342, -3.336375036156643733E-15 ) ) ;
#14460=CARTESIAN_POINT ( 'NONE',  ( -1.926257025242585782E-15, 196.1468750006145285, -31.45816453501075927 ) ) ;
#14480=CARTESIAN_POINT ( 'NONE',  ( -20.68320088531713452, 194.9994763905949924, -17.35526436380663284 ) ) ;
#14482=ORIENTED_EDGE ( 'NONE', *, *, #31242, .T. ) ;
#14508=CARTESIAN_POINT ( 'NONE',  ( -26.99999999999999645, 194.7500000012290400, 15.58845726811991561 ) ) ;
#14564=CARTESIAN_POINT ( 'NONE',  ( 7.234628195640322446, 198.4450961906613600, 26.99999999999999645 ) ) ;
#14584=CARTESIAN_POINT ( 'NONE',  ( 13.50000000000001421, 197.5625000012290400, 23.38268590217984055 ) ) ;
#14597=VECTOR ( 'NONE', #10150, 1000.000000000000000 ) ;
#14604=( BOUNDED_CURVE ( )  B_SPLINE_CURVE ( 2, ( #24705, #36257, #21871, #34167, #25820, #22803, #37367, #5530, #28656 ),
 .UNSPECIFIED., .F., .F. ) 
 B_SPLINE_CURVE_WITH_KNOTS ( ( 3, 2, 2, 2, 3 ),
 ( 0.5625000000000000000, 0.5694444444444444198, 0.5833333333333333703, 0.5972222222222222099, 0.6041666666666667407 ),
 .UNSPECIFIED. ) 
 CURVE ( )  GEOMETRIC_REPRESENTATION_ITEM ( )  RATIONAL_B_SPLINE_CURVE ( ( 0.9330127018922194093, 0.9330127018922194093, 1.000000000000000000, 0.8660254037844387076, 1.000000000000000000, 0.8660254037844387076, 1.000000000000000000, 0.9330127018922187432, 0.9330127018922192983 ) ) 
 REPRESENTATION_ITEM ( '' )  );
#14616=EDGE_LOOP ( 'NONE', ( #22188, #5446, #5222, #37210 ) ) ;
#14624=EDGE_LOOP ( 'NONE', ( #24486, #6390, #8293, #3897 ) ) ;
#14626=CARTESIAN_POINT ( 'NONE',  ( -27.24356964374999990, 198.8656250006145569, -15.72908226750537786 ) ) ;
#14647=CARTESIAN_POINT ( 'NONE',  ( -1.926257025242585782E-15, 195.2468750006145513, -31.45816453501075927 ) ) ;
#14664=CARTESIAN_POINT ( 'NONE',  ( 27.24356964374999635, 197.4218750006145342, -15.72908226750539029 ) ) ;
#14670=CARTESIAN_POINT ( 'NONE',  ( -7.234628195640302017, 195.5924038105676743, 27.00000000000000711 ) ) ;
#14693=CARTESIAN_POINT ( 'NONE',  ( -1.926257025242585782E-15, 198.7906250006145399, -31.45816453501076637 ) ) ;
#14776=CARTESIAN_POINT ( 'NONE',  ( -1.909035429704832693E-15, 195.9500000012290002, -31.17691453623979214 ) ) ;
#14789=CARTESIAN_POINT ( 'NONE',  ( 1.120210788295102201E-13, 196.8500000012290343, -27.00000000000000711 ) ) ;
#14796=CARTESIAN_POINT ( 'NONE',  ( 0.000000000000000000, 200.0000000000000000, 0.000000000000000000 ) ) ;
#14819=CARTESIAN_POINT ( 'NONE',  ( -13.62178482187500528, 198.8281250006145342, -23.59362340125807123 ) ) ;
#14838=CARTESIAN_POINT ( 'NONE',  ( 7.234628195640269155, 195.1825961894323598, 27.00000000000003197 ) ) ;
#14840=CARTESIAN_POINT ( 'NONE',  ( -1.926257025242585782E-15, 196.5968750006145456, -31.45816453501075927 ) ) ;
#14841=DIRECTION ( 'NONE',  ( -0.000000000000000000, -1.000000000000000000, -0.000000000000000000 ) ) ;
#14856=CARTESIAN_POINT ( 'NONE',  ( 27.24356964374999635, 197.8718750006145513, -15.72908226750539029 ) ) ;
#14883=CARTESIAN_POINT ( 'NONE',  ( -13.62178482187500528, 199.7281250006145399, -23.59362340125807123 ) ) ;
#14887=DIRECTION ( 'NONE',  ( 0.000000000000000000, 0.000000000000000000, -1.000000000000000000 ) ) ;
#14893=ORIENTED_EDGE ( 'NONE', *, *, #10865, .T. ) ;
#14896=CARTESIAN_POINT ( 'NONE',  ( 27.00000000000001421, 197.4875000000000114, 15.58845726811988897 ) ) ;
#14900=CARTESIAN_POINT ( 'NONE',  ( 26.99999999999999645, 198.9124999999999943, -15.58845726811990495 ) ) ;
#14936=( BOUNDED_CURVE ( )  B_SPLINE_CURVE ( 2, ( #17795, #9071, #29338, #23474, #12091, #14945, #3376, #35209, #24727 ),
 .UNSPECIFIED., .F., .F. ) 
 B_SPLINE_CURVE_WITH_KNOTS ( ( 3, 2, 2, 2, 3 ),
 ( 0.6041666666666667407, 0.6111111111111111605, 0.6250000000000000000, 0.6388888888888888395, 0.6458333333333333703 ),
 .UNSPECIFIED. ) 
 CURVE ( )  GEOMETRIC_REPRESENTATION_ITEM ( )  RATIONAL_B_SPLINE_CURVE ( ( 0.9330127018922192983, 0.9330127018922198534, 1.000000000000000000, 0.8660254037844387076, 1.000000000000000000, 0.8660254037844387076, 1.000000000000000000, 0.9330127018922187432, 0.9330127018922192983 ) ) 
 REPRESENTATION_ITEM ( '' )  );
#14945=CARTESIAN_POINT ( 'NONE',  ( 27.00000000000001421, 196.5875000000000341, 15.58845726811988897 ) ) ;
#14961=CARTESIAN_POINT ( 'NONE',  ( 27.00000000000000355, 195.3875000012290286, -3.306546357697854128E-15 ) ) ;
#14975=CARTESIAN_POINT ( 'NONE',  ( -26.99999999999999645, 199.1375000000000171, 15.58845726811991561 ) ) ;
#14979=CARTESIAN_POINT ( 'NONE',  ( -27.24356964374999990, 195.3218750006145399, -15.72908226750537786 ) ) ;
#15000=CARTESIAN_POINT ( 'NONE',  ( -27.24356964374999990, 197.9656250006145228, -15.72908226750537786 ) ) ;
#15025=CARTESIAN_POINT ( 'NONE',  ( -13.62178482187498396, 194.9843750006145626, 23.59362340125808188 ) ) ;
#15043=CARTESIAN_POINT ( 'NONE',  ( -1.926257025242585782E-15, 198.8468750006145740, -31.45816453501075927 ) ) ;
#15052=AXIS2_PLACEMENT_3D ( 'NONE', #27609, #1641, #24762 ) ;
#15069=CARTESIAN_POINT ( 'NONE',  ( -1.926257025242585782E-15, 199.2406250006145285, -31.45816453501076637 ) ) ;
#15087=ORIENTED_EDGE ( 'NONE', *, *, #22356, .F. ) ;
#15123=CARTESIAN_POINT ( 'NONE',  ( 26.99999999999999645, 198.5750000012290570, -15.58845726811990495 ) ) ;
#15166=EDGE_CURVE ( 'NONE', #24000, #27477, #29855, .T. ) ;
#15168=CARTESIAN_POINT ( 'NONE',  ( 27.24356964374999635, 196.0718750006145683, -15.72908226750539029 ) ) ;
#15178=CARTESIAN_POINT ( 'NONE',  ( 7.234628195640309123, 198.9674038105676743, -27.00000000000000711 ) ) ;
#15180=CARTESIAN_POINT ( 'NONE',  ( -1.926257025242585782E-15, 197.0468750006145342, -31.45816453501076637 ) ) ;
#15188=DIRECTION ( 'NONE',  ( 0.000000000000000000, 0.000000000000000000, -1.000000000000000000 ) ) ;
#15189=VERTEX_POINT ( 'NONE', #15368 ) ;
#15192=CARTESIAN_POINT ( 'NONE',  ( 13.62178482187501416, 197.7031250006145342, 23.59362340125806767 ) ) ;
#15193=EDGE_CURVE ( 'NONE', #10170, #15189, #33394, .T. ) ;
#15199=EDGE_CURVE ( 'NONE', #1318, #22836, #36165, .T. ) ;
#15201=CARTESIAN_POINT ( 'NONE',  ( 7.234628195640322446, 196.9825961894323427, 26.99999999999999645 ) ) ;
#15203=ORIENTED_EDGE ( 'NONE', *, *, #20272, .F. ) ;
#15207=ADVANCED_FACE ( 'NONE', ( #35820 ), #3612, .T. ) ;
#15217=CARTESIAN_POINT ( 'NONE',  ( -13.62178482187500528, 198.3781250006145171, -23.59362340125807123 ) ) ;
#15232=CARTESIAN_POINT ( 'NONE',  ( 27.24356964375000700, 198.6968750006145115, 15.72908226750537075 ) ) ;
#15258=CARTESIAN_POINT ( 'NONE',  ( -27.24356964374999990, 199.8218750006145399, -15.72908226750537786 ) ) ;
#15270=CARTESIAN_POINT ( 'NONE',  ( -4.694659320240884604E-14, 197.4124999999999943, 27.00000000000000000 ) ) ;
#15274=CARTESIAN_POINT ( 'NONE',  ( -13.50000000000000533, 199.4750000000000227, -23.38268590217984411 ) ) ;
#15289=PRODUCT_DEFINITION ( 'UNKNOWN', '', #22658, #34990 ) ;
#15318=AXIS2_PLACEMENT_3D ( 'NONE', #11319, #8115, #17387 ) ;
#15329=VERTEX_POINT ( 'NONE', #26918 ) ;
#15356=AXIS2_PLACEMENT_3D ( 'NONE', #11059, #34547, #16942 ) ;
#15357=CARTESIAN_POINT ( 'NONE',  ( -27.24356964374999635, 196.2968750006145342, 15.72908226750539384 ) ) ;
#15368=CARTESIAN_POINT ( 'NONE',  ( -20.86978604919638869, 194.8026013911397456, -17.51182792271053046 ) ) ;
#15370=CARTESIAN_POINT ( 'NONE',  ( -27.24356964374999279, 197.1968750006145115, 15.72908226750539384 ) ) ;
#15382=CARTESIAN_POINT ( 'NONE',  ( -13.62178482187498396, 197.6281250006145171, 23.59362340125808188 ) ) ;
#15411=CARTESIAN_POINT ( 'NONE',  ( -1.926257025242585782E-15, 197.4406250006145740, -31.45816453501075927 ) ) ;
#15412=CARTESIAN_POINT ( 'NONE',  ( 3.061616997868383043E-15, 200.0000000000000000, 25.00000000000000000 ) ) ;
#15417=DIRECTION ( 'NONE',  ( -0.000000000000000000, -1.000000000000000000, -0.000000000000000000 ) ) ;
#15434=DIRECTION ( 'NONE',  ( 0.000000000000000000, 1.000000000000000000, 0.000000000000000000 ) ) ;
#15449=CARTESIAN_POINT ( 'NONE',  ( -27.24356964375000345, 197.0656250006145171, -15.72908226750537786 ) ) ;
#15464=CARTESIAN_POINT ( 'NONE',  ( -27.24356964375000345, 199.8031250006145285, 0.000000000000000000 ) ) ;
#15465=CARTESIAN_POINT ( 'NONE',  ( -26.99999999999998934, 199.1375000000000171, 15.58845726811991561 ) ) ;
#15544=CARTESIAN_POINT ( 'NONE',  ( 7.234628195640318005, 199.0799038117967541, -26.99999999999999645 ) ) ;
#15546=CARTESIAN_POINT ( 'NONE',  ( -27.24356964375000345, 196.2593750006145399, 0.000000000000000000 ) ) ;
#15558=CARTESIAN_POINT ( 'NONE',  ( 27.24356964374999279, 196.9718750006145456, -15.72908226750539207 ) ) ;
#15566=CARTESIAN_POINT ( 'NONE',  ( -27.00000000000000355, 199.6625000012290343, 0.000000000000000000 ) ) ;
#15570=CARTESIAN_POINT ( 'NONE',  ( -27.24356964374999635, 197.5906250006145228, 15.72908226750539384 ) ) ;
#15595=CARTESIAN_POINT ( 'NONE',  ( 27.24356964374999635, 197.8156250006145171, -15.72908226750539029 ) ) ;
#15622=EDGE_CURVE ( 'NONE', #32805, #13180, #17760, .T. ) ;
#15627=CARTESIAN_POINT ( 'NONE',  ( -7.234628195640302017, 198.2924038105676630, 27.00000000000000711 ) ) ;
#15636=CARTESIAN_POINT ( 'NONE',  ( -13.62178482187500528, 197.9281250006145569, -23.59362340125807123 ) ) ;
#15648=( BOUNDED_CURVE ( )  B_SPLINE_CURVE ( 2, ( #11620, #17322, #34743, #17509, #20358, #28494, #3089, #2537, #11069 ),
 .UNSPECIFIED., .F., .F. ) 
 B_SPLINE_CURVE_WITH_KNOTS ( ( 3, 2, 2, 2, 3 ),
 ( 0.4375000000000000000, 0.4444444444444444198, 0.4583333333333333148, 0.4722222222222222099, 0.4791666666666666852 ),
 .UNSPECIFIED. ) 
 CURVE ( )  GEOMETRIC_REPRESENTATION_ITEM ( )  RATIONAL_B_SPLINE_CURVE ( ( 0.9330127018922194093, 0.9330127018922194093, 1.000000000000000000, 0.8660254037844387076, 1.000000000000000000, 0.8660254037844387076, 1.000000000000000000, 0.9330127018922190762, 0.9330127018922194093 ) ) 
 REPRESENTATION_ITEM ( '' )  );
#15654=CARTESIAN_POINT ( 'NONE',  ( -27.00000000000000355, 199.0999999999999943, 0.000000000000000000 ) ) ;
#15655=EDGE_LOOP ( 'NONE', ( #6072, #2294, #1188 ) ) ;
#15659=ORIENTED_EDGE ( 'NONE', *, *, #33716, .T. ) ;
#15662=CARTESIAN_POINT ( 'NONE',  ( -27.00000000000000355, 199.2125000012290457, 0.000000000000000000 ) ) ;
#15666=CARTESIAN_POINT ( 'NONE',  ( 0.000000000000000000, 200.0000000000000000, -27.00000000000000355 ) ) ;
#15718=EDGE_CURVE ( 'NONE', #19052, #37126, #6953, .T. ) ;
#15729=CARTESIAN_POINT ( 'NONE',  ( -13.49999999999998401, 197.8249999999999886, 23.38268590217985476 ) ) ;
#15743=CARTESIAN_POINT ( 'NONE',  ( 3.253724281355069334E-15, 199.5500000012290513, -27.00000000000000000 ) ) ;
#15747=CARTESIAN_POINT ( 'NONE',  ( 27.24356964374999279, 198.3218750006145399, -15.72908226750539207 ) ) ;
#15761=CARTESIAN_POINT ( 'NONE',  ( -13.62178482187500528, 197.4781250006145399, -23.59362340125807123 ) ) ;
#15774=CARTESIAN_POINT ( 'NONE',  ( 7.234628195640363302, 195.4799038117967029, -26.99999999999996803 ) ) ;
#15788=CARTESIAN_POINT ( 'NONE',  ( 5.778771075727756162E-15, 198.5656250006145171, 31.45816453501075927 ) ) ;
#15801=ORIENTED_EDGE ( 'NONE', *, *, #8322, .T. ) ;
#15823=CARTESIAN_POINT ( 'NONE',  ( 13.62178482187499640, 196.9531250006145342, -23.59362340125807123 ) ) ;
#15840=CARTESIAN_POINT ( 'NONE',  ( 5.727106289114498080E-15, 196.5125000000000171, 31.17691453623979214 ) ) ;
#15871=CARTESIAN_POINT ( 'NONE',  ( -7.234628195640316228, 195.9700961906613372, -27.00000000000000000 ) ) ;
#15898=ORIENTED_EDGE ( 'NONE', *, *, #28459, .T. ) ;
#15917=CARTESIAN_POINT ( 'NONE',  ( 27.00000000000000355, 196.1750000000000114, -3.306546357697854128E-15 ) ) ;
#15939=CARTESIAN_POINT ( 'NONE',  ( 27.24356964374999279, 197.4218750006145342, -15.72908226750539207 ) ) ;
#15951=CARTESIAN_POINT ( 'NONE',  ( -27.24356964374999635, 197.1406250006145058, 15.72908226750539384 ) ) ;
#15967=CARTESIAN_POINT ( 'NONE',  ( 13.49999999999999645, 199.4000000000000341, -23.38268590217984766 ) ) ;
#15977=CARTESIAN_POINT ( 'NONE',  ( 27.24356964375000700, 199.0906250006145228, 15.72908226750537075 ) ) ;
#15982=ADVANCED_FACE ( 'NONE', ( #32667, #18280 ), #29824, .T. ) ;
#16005=CARTESIAN_POINT ( 'NONE',  ( 26.99999999999999645, 195.8750000012290400, -15.58845726811990495 ) ) ;
#16016=CARTESIAN_POINT ( 'NONE',  ( -27.24356964375000345, 196.6531250006145513, 0.000000000000000000 ) ) ;
#16031=CARTESIAN_POINT ( 'NONE',  ( -13.50000000000000533, 198.5749999999999886, -23.38268590217984411 ) ) ;
#16039=CARTESIAN_POINT ( 'NONE',  ( -1.045839947578415010E-13, 196.5125000000000455, 27.00000000000000355 ) ) ;
#16047=CARTESIAN_POINT ( 'NONE',  ( 0.000000000000000000, 0.000000000000000000, 0.000000000000000000 ) ) ;
#16057=ORIENTED_EDGE ( 'NONE', *, *, #7625, .T. ) ;
#16090=VECTOR ( 'NONE', #32509, 1000.000000000000000 ) ;
#16093=CARTESIAN_POINT ( 'NONE',  ( -27.00000000000000355, 199.5124999999999886, -15.58845726811989429 ) ) ;
#16124=CARTESIAN_POINT ( 'NONE',  ( 13.62178482187499640, 195.6593750006145456, -23.59362340125807123 ) ) ;
#16135=CARTESIAN_POINT ( 'NONE',  ( 27.24356964375000700, 195.9406250006145456, 15.72908226750537075 ) ) ;
#16145=( BOUNDED_CURVE ( )  B_SPLINE_CURVE ( 2, ( #20959, #32120, #34964, #14508, #19708, #8822, #17547 ),
 .UNSPECIFIED., .F., .F. ) 
 B_SPLINE_CURVE_WITH_KNOTS ( ( 3, 2, 2, 3 ),
 ( 0.8958333333333333703, 0.9027777777777777901, 0.9166666666666666297, 0.9258785558287927486 ),
 .UNSPECIFIED. ) 
 CURVE ( )  GEOMETRIC_REPRESENTATION_ITEM ( )  RATIONAL_B_SPLINE_CURVE ( ( 0.9330127018922192983, 0.9330127018922198534, 1.000000000000000000, 0.8660254037844387076, 1.000000000000000000, 0.9111405425767590271, 0.9401542252352144136 ) ) 
 REPRESENTATION_ITEM ( '' )  );
#16149=DIRECTION ( 'NONE',  ( 0.000000000000000000, 0.000000000000000000, -1.000000000000000000 ) ) ;
#16154=CARTESIAN_POINT ( 'NONE',  ( 7.234628195640318005, 199.4174038105677198, -26.99999999999999645 ) ) ;
#16158=DIRECTION ( 'NONE',  ( -0.000000000000000000, -1.000000000000000000, -0.000000000000000000 ) ) ;
#16162=CARTESIAN_POINT ( 'NONE',  ( 27.24356964375000700, 196.3906250006145058, 15.72908226750537075 ) ) ;
#16200=AXIS2_PLACEMENT_3D ( 'NONE', #36555, #11712, #17416 ) ;
#16201=CARTESIAN_POINT ( 'NONE',  ( 27.24356964374999279, 198.7156250006145513, -15.72908226750539207 ) ) ;
#16202=CARTESIAN_POINT ( 'NONE',  ( -27.24356964374999635, 197.1968750006145115, 15.72908226750539384 ) ) ;
#16216=CARTESIAN_POINT ( 'NONE',  ( -27.00000000000000355, 197.2624999999999886, -15.58845726811989429 ) ) ;
#16217=ORIENTED_EDGE ( 'NONE', *, *, #19583, .T. ) ;
#16223=CARTESIAN_POINT ( 'NONE',  ( -7.234628195640302017, 199.3049038117967200, 27.00000000000000711 ) ) ;
#16232=SURFACE_SIDE_STYLE ('',( #16418 ) ) ;
#16269=CARTESIAN_POINT ( 'NONE',  ( 1.069080835302379631E-14, 198.7624999999999886, 27.00000000000000000 ) ) ;
#16274=EDGE_LOOP ( 'NONE', ( #25786, #19217, #28502 ) ) ;
#16283=AXIS2_PLACEMENT_3D ( 'NONE', #36912, #28388, #14185 ) ;
#16293=CARTESIAN_POINT ( 'NONE',  ( 0.000000000000000000, 200.0000000000000000, -27.00000000000000355 ) ) ;
#16299=ORIENTED_EDGE ( 'NONE', *, *, #7794, .F. ) ;
#16321=CARTESIAN_POINT ( 'NONE',  ( -27.00000000000000355, 198.7625000012290286, 0.000000000000000000 ) ) ;
#16336=CARTESIAN_POINT ( 'NONE',  ( 27.00000000000001421, 197.9375000000000284, 15.58845726811988897 ) ) ;
#16342=DIRECTION ( 'NONE',  ( -0.000000000000000000, -1.000000000000000000, -0.000000000000000000 ) ) ;
#16344=CARTESIAN_POINT ( 'NONE',  ( 27.24356964375000345, 195.5281250006145228, -3.336375036156643733E-15 ) ) ;
#16387=CARTESIAN_POINT ( 'NONE',  ( -27.24356964375000345, 195.7531250006145456, 0.000000000000000000 ) ) ;
#16388=CARTESIAN_POINT ( 'NONE',  ( -27.24356964374999635, 198.0968750006145456, 15.72908226750539384 ) ) ;
#16391=CARTESIAN_POINT ( 'NONE',  ( -26.99999999999999645, 195.0875000000000341, 15.58845726811991561 ) ) ;
#16403=CARTESIAN_POINT ( 'NONE',  ( -1.909035429704832693E-15, 198.0875000000000341, -31.17691453623979214 ) ) ;
#16417=EDGE_CURVE ( 'NONE', #36062, #4383, #6663, .T. ) ;
#16418=SURFACE_STYLE_FILL_AREA ( #22477 ) ;
#16467=CARTESIAN_POINT ( 'NONE',  ( -1.045839947578415010E-13, 195.7250000012290343, 27.00000000000000355 ) ) ;
#16509=CARTESIAN_POINT ( 'NONE',  ( 5.727106289114498080E-15, 198.4250000012290229, 31.17691453623979214 ) ) ;
#16531=CARTESIAN_POINT ( 'NONE',  ( 27.24356964375000345, 195.0781250006145342, -3.336375036156643733E-15 ) ) ;
#16536=AXIS2_PLACEMENT_3D ( 'NONE', #34366, #33817, #16758 ) ;
#16548=VERTEX_POINT ( 'NONE', #6854 ) ;
#16551=CARTESIAN_POINT ( 'NONE',  ( -27.00000000000000355, 199.9625000000000057, -15.58845726811989429 ) ) ;
#16560=CARTESIAN_POINT ( 'NONE',  ( 27.00000000000000355, 195.8375000012290457, -3.306546357697854128E-15 ) ) ;
#16572=CARTESIAN_POINT ( 'NONE',  ( 5.778771075727756162E-15, 194.9656250006145797, 31.45816453501076637 ) ) ;
#16573=CARTESIAN_POINT ( 'NONE',  ( 27.24356964375000700, 198.2468750006145513, 15.72908226750537075 ) ) ;
#16582=EDGE_LOOP ( 'NONE', ( #15087, #33694, #10944, #19984 ) ) ;
#16591=CARTESIAN_POINT ( 'NONE',  ( -27.24356964374999990, 199.8218750006145399, -15.72908226750537786 ) ) ;
#16646=ORIENTED_EDGE ( 'NONE', *, *, #8322, .F. ) ;
#16681=CARTESIAN_POINT ( 'NONE',  ( -1.045839947578415010E-13, 196.1750000012290229, 27.00000000000000355 ) ) ;
#16696=CARTESIAN_POINT ( 'NONE',  ( 27.00000000000000355, 199.4375000012290400, -3.306546357697854128E-15 ) ) ;
#16718=LINE ( 'NONE', #13872, #35718 ) ;
#16719=CARTESIAN_POINT ( 'NONE',  ( -27.24356964374999990, 196.1656250006145399, -15.72908226750537786 ) ) ;
#16754=CARTESIAN_POINT ( 'NONE',  ( -13.62178482187500528, 196.1281250006145171, -23.59362340125807123 ) ) ;
#16755=CARTESIAN_POINT ( 'NONE',  ( -13.62178482187500528, 197.9843750006145626, -23.59362340125807123 ) ) ;
#16758=DIRECTION ( 'NONE',  ( 0.000000000000000000, 0.000000000000000000, -1.000000000000000000 ) ) ;
#16772=CARTESIAN_POINT ( 'NONE',  ( 5.727106289114498080E-15, 195.6125000000000398, 31.17691453623979214 ) ) ;
#16798=EDGE_CURVE ( 'NONE', #32409, #32329, #33384, .T. ) ;
#16799=ORIENTED_EDGE ( 'NONE', *, *, #29045, .F. ) ;
#16821=PRODUCT ( 'Cylinder', 'Cylinder', '', ( #6962 ) ) ;
#16871=CARTESIAN_POINT ( 'NONE',  ( -13.62178482187500528, 195.2843750006145456, -23.59362340125807123 ) ) ;
#16882=CARTESIAN_POINT ( 'NONE',  ( 13.50000000000001421, 199.3625000012290513, 23.38268590217984055 ) ) ;
#16903=CARTESIAN_POINT ( 'NONE',  ( -27.24356964375000345, 195.3031250006145285, 0.000000000000000000 ) ) ;
#16929=EDGE_LOOP ( 'NONE', ( #27431, #19818, #11756, #19385 ) ) ;
#16941=CARTESIAN_POINT ( 'NONE',  ( -1.926257025242585782E-15, 198.3968750006145285, -31.45816453501075927 ) ) ;
#16942=DIRECTION ( 'NONE',  ( 0.000000000000000000, 0.000000000000000000, -1.000000000000000000 ) ) ;
#16951=CARTESIAN_POINT ( 'NONE',  ( -27.00000000000000355, 195.9500000000000171, 0.000000000000000000 ) ) ;
#16957=CARTESIAN_POINT ( 'NONE',  ( -13.49999999999998401, 195.5749999999999886, 23.38268590217985476 ) ) ;
#16960=ORIENTED_EDGE ( 'NONE', *, *, #36975, .F. ) ;
#17006=CARTESIAN_POINT ( 'NONE',  ( -13.49999999999998401, 196.5875000012290457, 23.38268590217985476 ) ) ;
#17032=DIRECTION ( 'NONE',  ( -0.000000000000000000, -1.000000000000000000, -0.000000000000000000 ) ) ;
#17063=CARTESIAN_POINT ( 'NONE',  ( 13.50000000000001421, 198.0125000012290286, 23.38268590217984055 ) ) ;
#17077=FACE_OUTER_BOUND ( 'NONE', #16929, .T. ) ;
#17115=CARTESIAN_POINT ( 'NONE',  ( -20.74539548491456387, 194.9526013907998276, -17.40745275905709377 ) ) ;
#17128=CARTESIAN_POINT ( 'NONE',  ( 26.99999999999999645, 195.3125000000000000, -15.58845726811990495 ) ) ;
#17129=CARTESIAN_POINT ( 'NONE',  ( 5.778771075727756162E-15, 196.3718750006145513, 31.45816453501075927 ) ) ;
#17147=CARTESIAN_POINT ( 'NONE',  ( 5.727106289114498080E-15, 196.0625000000000000, 31.17691453623979214 ) ) ;
#17153=DIRECTION ( 'NONE',  ( 0.000000000000000000, 0.000000000000000000, -1.000000000000000000 ) ) ;
#17215=AXIS2_PLACEMENT_3D ( 'NONE', #16047, #4651, #19645 ) ;
#17216=VERTEX_POINT ( 'NONE', #12304 ) ;
#17224=DIRECTION ( 'NONE',  ( 0.000000000000000000, 1.000000000000000000, 0.000000000000000000 ) ) ;
#17228=CARTESIAN_POINT ( 'NONE',  ( -13.49999999999998401, 197.3750000000000284, 23.38268590217985476 ) ) ;
#17248=CARTESIAN_POINT ( 'NONE',  ( 13.50000000000001421, 196.6625000012290343, 23.38268590217984055 ) ) ;
#17279=CARTESIAN_POINT ( 'NONE',  ( -27.24356964375000345, 198.5093750006145399, 0.000000000000000000 ) ) ;
#17289=AXIS2_PLACEMENT_3D ( 'NONE', #8371, #19569, #14059 ) ;
#17290=CARTESIAN_POINT ( 'NONE',  ( -1.926257025242585782E-15, 199.6906250006145456, -31.45816453501075927 ) ) ;
#17294=CYLINDRICAL_SURFACE ( 'NONE', #19220, 27.00000000000000355 ) ;
#17305=( BOUNDED_CURVE ( )  B_SPLINE_CURVE ( 2, ( #1258, #12827, #27606, #18910, #9983, #24395, #36688, #15871, #10726 ),
 .UNSPECIFIED., .F., .F. ) 
 B_SPLINE_CURVE_WITH_KNOTS ( ( 3, 2, 2, 2, 3 ),
 ( 0.6458333333333333703, 0.6527777777777777901, 0.6666666666666666297, 0.6805555555555555802, 0.6875000000000000000 ),
 .UNSPECIFIED. ) 
 CURVE ( )  GEOMETRIC_REPRESENTATION_ITEM ( )  RATIONAL_B_SPLINE_CURVE ( ( 0.9330127018922192983, 0.9330127018922198534, 1.000000000000000000, 0.8660254037844387076, 1.000000000000000000, 0.8660254037844387076, 1.000000000000000000, 0.9330127018922194093, 0.9330127018922194093 ) ) 
 REPRESENTATION_ITEM ( '' )  );
#17311=CARTESIAN_POINT ( 'NONE',  ( 27.24356964375000345, 196.4843750006145626, -3.336375036156643733E-15 ) ) ;
#17322=CARTESIAN_POINT ( 'NONE',  ( 7.234628195640309123, 197.2799038117966859, -27.00000000000000711 ) ) ;
#17324=EDGE_LOOP ( 'NONE', ( #349, #33414, #20551, #36663 ) ) ;
#17330=CARTESIAN_POINT ( 'NONE',  ( -13.49999999999998401, 196.0250000000000057, 23.38268590217985476 ) ) ;
#17336=CARTESIAN_POINT ( 'NONE',  ( 1.069080835302379631E-14, 196.9624999999999773, 27.00000000000000000 ) ) ;
#17362=CARTESIAN_POINT ( 'NONE',  ( -27.24356964374999279, 199.3906250006145342, 15.72908226750539384 ) ) ;
#17369=CARTESIAN_POINT ( 'NONE',  ( -27.00000000000000355, 197.8250000012290570, -15.58845726811989429 ) ) ;
#17380=CARTESIAN_POINT ( 'NONE',  ( -26.99999999999999645, 196.5500000012290513, 15.58845726811991561 ) ) ;
#17387=DIRECTION ( 'NONE',  ( 0.000000000000000000, 0.000000000000000000, 1.000000000000000000 ) ) ;
#17394=VECTOR ( 'NONE', #5958, 999.9999999999998863 ) ;
#17410=CARTESIAN_POINT ( 'NONE',  ( -27.00000000000000355, 196.9250000012290229, -15.58845726811989429 ) ) ;
#17416=DIRECTION ( 'NONE',  ( 0.000000000000000000, 0.000000000000000000, -1.000000000000000000 ) ) ;
#17436=CARTESIAN_POINT ( 'NONE',  ( -27.00000000000000355, 195.6125000012290513, 0.000000000000000000 ) ) ;
#17451=CARTESIAN_POINT ( 'NONE',  ( 7.234628195640322446, 196.6450961906613770, 26.99999999999999645 ) ) ;
#17466=CARTESIAN_POINT ( 'NONE',  ( 27.24356964375000345, 199.6343750006145399, -3.336375036156643733E-15 ) ) ;
#17469=VERTEX_POINT ( 'NONE', #20787 ) ;
#17479=CARTESIAN_POINT ( 'NONE',  ( -27.24356964374999990, 198.4156250006145399, -15.72908226750537786 ) ) ;
#17499=CARTESIAN_POINT ( 'NONE',  ( 27.24356964375000345, 196.0343750006145456, -3.336375036156643733E-15 ) ) ;
#17509=CARTESIAN_POINT ( 'NONE',  ( 26.99999999999999645, 197.2250000012290343, -15.58845726811990495 ) ) ;
#17518=CARTESIAN_POINT ( 'NONE',  ( -13.62178482187500528, 197.0843750006145285, -23.59362340125807123 ) ) ;
#17521=ORIENTED_EDGE ( 'NONE', *, *, #16798, .F. ) ;
#17547=CARTESIAN_POINT ( 'NONE',  ( -20.68320086892770604, 194.6619763917542798, -17.35526438333879540 ) ) ;
#17562=CARTESIAN_POINT ( 'NONE',  ( 7.234628195640309123, 197.6174038105676516, -27.00000000000000711 ) ) ;
#17602=CARTESIAN_POINT ( 'NONE',  ( 1.069080835302379631E-14, 198.4250000012290229, 27.00000000000000000 ) ) ;
#17606=CARTESIAN_POINT ( 'NONE',  ( 5.438367727407757775E-14, 198.5374999999999943, -27.00000000000000355 ) ) ;
#17608=ORIENTED_EDGE ( 'NONE', *, *, #32700, .T. ) ;
#17627=CARTESIAN_POINT ( 'NONE',  ( 27.00000000000000355, 196.2875000012290343, -3.306546357697854128E-15 ) ) ;
#17644=CARTESIAN_POINT ( 'NONE',  ( 27.00000000000000355, 194.9375000012290400, -3.306546357697854128E-15 ) ) ;
#17648=DIRECTION ( 'NONE',  ( 0.000000000000000000, 0.000000000000000000, -1.000000000000000000 ) ) ;
#17667=ORIENTED_EDGE ( 'NONE', *, *, #18504, .T. ) ;
#17668=CARTESIAN_POINT ( 'NONE',  ( 27.24356964375000345, 199.1281250006145171, -3.336375036156643733E-15 ) ) ;
#17688=CARTESIAN_POINT ( 'NONE',  ( -27.24356964374999990, 195.7718750006145569, -15.72908226750537786 ) ) ;
#17689=CARTESIAN_POINT ( 'NONE',  ( 26.99999999999999645, 198.1250000012290400, -15.58845726811990495 ) ) ;
#17690=CARTESIAN_POINT ( 'NONE',  ( -13.50000000000000533, 198.5749999999999886, -23.38268590217984411 ) ) ;
#17703=CARTESIAN_POINT ( 'NONE',  ( -27.24356964374999635, 198.5468750006145626, 15.72908226750539384 ) ) ;
#17723=ORIENTED_EDGE ( 'NONE', *, *, #27451, .F. ) ;
#17730=CARTESIAN_POINT ( 'NONE',  ( 13.62178482187501416, 199.5031250006145456, 23.59362340125806767 ) ) ;
#17736=CARTESIAN_POINT ( 'NONE',  ( 0.000000000000000000, 200.0000000000000000, 0.000000000000000000 ) ) ;
#17744=PRODUCT_DEFINITION_SHAPE ( 'NONE', 'NONE',  #15289 ) ;
#17749=CARTESIAN_POINT ( 'NONE',  ( 27.00000000000000355, 199.7750000000000057, -3.306546357697854128E-15 ) ) ;
#17760=LINE ( 'NONE', #2781, #6074 ) ;
#17790=CARTESIAN_POINT ( 'NONE',  ( -20.86978606573367045, 194.8588513912095266, -17.51182790300216752 ) ) ;
#17795=CARTESIAN_POINT ( 'NONE',  ( 1.120210788295102201E-13, 196.7375000000000398, -27.00000000000000711 ) ) ;
#17812=CARTESIAN_POINT ( 'NONE',  ( 13.49999999999999645, 195.4625000012290172, -23.38268590217984766 ) ) ;
#17818=EDGE_CURVE ( 'NONE', #17469, #26583, #27210, .T. ) ;
#17832=CARTESIAN_POINT ( 'NONE',  ( 1.069080835302379631E-14, 199.2125000000000057, 27.00000000000000000 ) ) ;
#17836=CARTESIAN_POINT ( 'NONE',  ( -27.24356964375000345, 195.8093750006145513, 0.000000000000000000 ) ) ;
#17842=DIRECTION ( 'NONE',  ( 1.000000000000000000, 0.000000000000000000, 0.000000000000000000 ) ) ;
#17844=FACE_BOUND ( 'NONE', #6577, .T. ) ;
#17847=CARTESIAN_POINT ( 'NONE',  ( 13.62178482187499640, 199.2593750006145399, -23.59362340125807123 ) ) ;
#17856=CARTESIAN_POINT ( 'NONE',  ( 5.778771075727756162E-15, 199.0156250006145342, 31.45816453501075927 ) ) ;
#17875=CARTESIAN_POINT ( 'NONE',  ( -7.234628195640302017, 198.8549038117967029, 27.00000000000000711 ) ) ;
#17877=CARTESIAN_POINT ( 'NONE',  ( -13.62178482187498396, 196.7843750006145456, 23.59362340125808188 ) ) ;
#17893=CARTESIAN_POINT ( 'NONE',  ( -1.926257025242585782E-15, 197.9468750006145399, -31.45816453501075927 ) ) ;
#17920=CARTESIAN_POINT ( 'NONE',  ( 27.24356964375000700, 199.5406250006145967, 15.72908226750537075 ) ) ;
#17977=DIRECTION ( 'NONE',  ( -0.000000000000000000, -1.000000000000000000, -0.000000000000000000 ) ) ;
#18001=CARTESIAN_POINT ( 'NONE',  ( 26.99999999999999645, 194.9750000012290343, -15.58845726811990495 ) ) ;
#18020=CARTESIAN_POINT ( 'NONE',  ( -13.62178482187500528, 196.6343750006145399, -23.59362340125807123 ) ) ;
#18029=DIRECTION ( 'NONE',  ( 0.000000000000000000, -0.000000000000000000, 1.000000000000000000 ) ) ;
#18034=VERTEX_POINT ( 'NONE', #9891 ) ;
#18044=AXIS2_PLACEMENT_3D ( 'NONE', #6718, #5962, #29646 ) ;
#18045=CARTESIAN_POINT ( 'NONE',  ( 13.62178482187501416, 199.0531250006145285, 23.59362340125806767 ) ) ;
#18053=CARTESIAN_POINT ( 'NONE',  ( 27.00000000000000355, 197.0749999999999886, -3.306546357697854128E-15 ) ) ;
#18070=CARTESIAN_POINT ( 'NONE',  ( -13.62178482187500528, 198.8281250006145342, -23.59362340125807123 ) ) ;
#18085=CARTESIAN_POINT ( 'NONE',  ( 13.62178482187501416, 197.3093750006145513, 23.59362340125806767 ) ) ;
#18111=CARTESIAN_POINT ( 'NONE',  ( 27.24356964374999279, 199.6156250006145285, -15.72908226750539207 ) ) ;
#18117=CARTESIAN_POINT ( 'NONE',  ( -27.00000000000000355, 199.6625000012290343, 0.000000000000000000 ) ) ;
#18142=CARTESIAN_POINT ( 'NONE',  ( 0.000000000000000000, 200.0000000000000000, 0.000000000000000000 ) ) ;
#18167=CARTESIAN_POINT ( 'NONE',  ( -4.694659320240884604E-14, 197.8625000000000114, 27.00000000000000000 ) ) ;
#18207=CARTESIAN_POINT ( 'NONE',  ( 13.50000000000001421, 198.9125000012290343, 23.38268590217984055 ) ) ;
#18209=CARTESIAN_POINT ( 'NONE',  ( 13.62178482187499640, 196.5593750006145513, -23.59362340125807123 ) ) ;
#18220=CARTESIAN_POINT ( 'NONE',  ( 27.00000000000001421, 198.8374999999999773, 15.58845726811988897 ) ) ;
#18222=CARTESIAN_POINT ( 'NONE',  ( -13.62178482187498396, 197.2343750006145626, 23.59362340125808188 ) ) ;
#18230=CARTESIAN_POINT ( 'NONE',  ( 1.120210788295102201E-13, 196.4000000012290741, -27.00000000000000711 ) ) ;
#18233=CARTESIAN_POINT ( 'NONE',  ( -13.62178482187500528, 196.5781250006145342, -23.59362340125807123 ) ) ;
#18256=CARTESIAN_POINT ( 'NONE',  ( -27.24356964374999990, 197.5156250006145626, -15.72908226750537786 ) ) ;
#18270=CARTESIAN_POINT ( 'NONE',  ( -27.24356964374999990, 198.4718750006145171, -15.72908226750537786 ) ) ;
#18280=FACE_BOUND ( 'NONE', #34728, .T. ) ;
#18299=CARTESIAN_POINT ( 'NONE',  ( -27.24356964375000345, 197.5531250006145285, 0.000000000000000000 ) ) ;
#18311=CYLINDRICAL_SURFACE ( 'NONE', #18411, 27.00000000000000355 ) ;
#18318=ORIENTED_EDGE ( 'NONE', *, *, #23982, .T. ) ;
#18338=EDGE_LOOP ( 'NONE', ( #33881, #31312, #21491, #11680 ) ) ;
#18342=FACE_OUTER_BOUND ( 'NONE', #33834, .T. ) ;
#18375=CARTESIAN_POINT ( 'NONE',  ( -27.00000000000000355, 194.6888594429640591, -9.827195528215911580 ) ) ;
#18391=CARTESIAN_POINT ( 'NONE',  ( -13.50000000000000533, 199.0250000000000057, -23.38268590217984411 ) ) ;
#18395=VECTOR ( 'NONE', #14841, 1000.000000000000000 ) ;
#18406=CARTESIAN_POINT ( 'NONE',  ( -20.74539548491456031, 194.7088513915494445, -17.40745275905709377 ) ) ;
#18408=CARTESIAN_POINT ( 'NONE',  ( 27.24356964375000700, 196.8968750006144717, 15.72908226750537075 ) ) ;
#18410=ORIENTED_EDGE ( 'NONE', *, *, #3630, .T. ) ;
#18411=AXIS2_PLACEMENT_3D ( 'NONE', #3887, #27012, #1039 ) ;
#18423=CARTESIAN_POINT ( 'NONE',  ( 5.778771075727756162E-15, 195.4156250006145399, 31.45816453501075927 ) ) ;
#18426=EDGE_CURVE ( 'NONE', #5428, #55, #30865, .T. ) ;
#18450=CARTESIAN_POINT ( 'NONE',  ( -1.926257025242585782E-15, 197.8906250006145342, -31.45816453501075927 ) ) ;
#18466=EDGE_CURVE ( 'NONE', #36062, #5775, #27857, .T. ) ;
#18491=CARTESIAN_POINT ( 'NONE',  ( -27.24356964375000345, 198.4156250006145399, -15.72908226750537786 ) ) ;
#18492=CARTESIAN_POINT ( 'NONE',  ( 27.24356964374999635, 199.6718750006145058, -15.72908226750539029 ) ) ;
#18504=EDGE_CURVE ( 'NONE', #26034, #11516, #1520, .T. ) ;
#18508=CARTESIAN_POINT ( 'NONE',  ( 0.000000000000000000, 200.0000000000000000, 0.000000000000000000 ) ) ;
#18509=CARTESIAN_POINT ( 'NONE',  ( -13.49999999999998401, 199.6250000000000284, 23.38268590217985476 ) ) ;
#18546=FACE_OUTER_BOUND ( 'NONE', #12515, .T. ) ;
#18599=CARTESIAN_POINT ( 'NONE',  ( 0.000000000000000000, 0.000000000000000000, 0.000000000000000000 ) ) ;
#18600=CARTESIAN_POINT ( 'NONE',  ( 7.234628195640322446, 199.3450961906613657, 26.99999999999999645 ) ) ;
#18604=CARTESIAN_POINT ( 'NONE',  ( 13.62178482187499640, 197.9093750006145456, -23.59362340125807123 ) ) ;
#18606=ORIENTED_EDGE ( 'NONE', *, *, #20272, .T. ) ;
#18617=CARTESIAN_POINT ( 'NONE',  ( 27.24356964375000700, 195.4906250006145001, 15.72908226750537075 ) ) ;
#18642=CARTESIAN_POINT ( 'NONE',  ( 13.62178482187499640, 199.2031250006145342, -23.59362340125807123 ) ) ;
#18677=CARTESIAN_POINT ( 'NONE',  ( -13.49999999999998401, 197.4875000012290229, 23.38268590217985476 ) ) ;
#18681=CARTESIAN_POINT ( 'NONE',  ( 27.24356964375000345, 197.7781250006145228, -3.336375036156643733E-15 ) ) ;
#18682=EDGE_CURVE ( 'NONE', #19052, #25162, #9277, .T. ) ;
#18691=ORIENTED_EDGE ( 'NONE', *, *, #7625, .F. ) ;
#18698=CARTESIAN_POINT ( 'NONE',  ( 26.99999999999999645, 196.6625000000000227, -15.58845726811990495 ) ) ;
#18703=ORIENTED_EDGE ( 'NONE', *, *, #5546, .F. ) ;
#18739=DIRECTION ( 'NONE',  ( -0.000000000000000000, -1.000000000000000000, 0.000000000000000000 ) ) ;
#18753=EDGE_LOOP ( 'NONE', ( #30518, #16799, #9120, #3993, #19005, #30918 ) ) ;
#18761=CARTESIAN_POINT ( 'NONE',  ( 27.00000000000000355, 194.9375000012290400, -3.306546357697854128E-15 ) ) ;
#18793=CARTESIAN_POINT ( 'NONE',  ( 27.24356964375000700, 197.7968750006145342, 15.72908226750537075 ) ) ;
#18805=CARTESIAN_POINT ( 'NONE',  ( 5.778771075727756162E-15, 197.2156250006145513, 31.45816453501075927 ) ) ;
#18813=( BOUNDED_SURFACE ( )  B_SPLINE_SURFACE ( 1, 2, ( 
 ( #12615, #24181, #665, #481, #26827, #32326, #17749, #12236, #34982, #3329, #18509, #30048, #6554, #12048, #15274, #21349, #6741, #857, #12428, #23997, #3894, #296, #21161, #15465, #15654, #32889, #27019, #11861, #9025, #14900, #23619, #9212, #1228, #27580, #30620, #4451, #21718, #7680, #16031, #13179, #21902, #1609, #36102, #30991, #1796, #36662, #27766, #33083, #33641, #5009, #12799, #16403, #27203, #27949, #24369, #24733, #12996, #10331, #36283, #30239, #35913, #30431, #33449, #24552, #1979, #19260, #4265, #7492, #33830, #19068, #4637, #7126, #33269, #16216, #10511, #13363, #21537, #30799, #10145, #24918, #36470, #7867, #9956, #7308, #10700, #22091, #4822, #13551, #18880, #18698, #25104, #22277, #19441, #15840, #27388, #1418, #8053, #36845, #28500, #2356, #11075, #2164, #11264, #61, #2722, #17147, #17330, #2543, #10888, #14110, #13929, #31909, #5377, #22461, #37398, #37217, #11628, #16772, #16957, #28873, #2908, #25662, #28318, #5562, #37029, #34008, #34196, #13747, #19629, #23203, #34751, #22650, #5197, #22834, #14480 ),
 ( #11448, #16591, #28683, #23015, #8794, #26033, #19816, #31536, #8242, #8423, #20366, #25478, #28135, #34382, #19992, #31351, #14297, #34565, #25850, #8605, #20175, #31723, #5751, #25293, #31175, #23953, #32093, #15043, #23574, #6125, #6699, #15232, #9357, #26214, #6321, #17703, #35119, #18270, #32278, #29052, #20550, #26591, #251, #9168, #20735, #3284, #3096, #12383, #438, #29243, #35301, #17893, #12003, #14856, #20928, #32467, #621, #6510, #29438, #3474, #21119, #11815, #812, #12190, #26782, #14664, #23762, #26405, #18085, #32658, #29626, #5939, #8979, #23385, #17518, #3661, #35495, #9545, #34934, #3782, #9296, #32028, #29945, #3973, #29372, #11942, #18020, #35622, #18209, #20868, #748, #3410, #29751, #23322, #35433, #15357, #15546, #24077, #26528, #12319, #6259, #15168, #9668, #20672, #34873, #23700, #26716, #559, #17836, #26911, #12125, #32407, #29565, #35243, #32220, #27104, #9481, #32785, #35057, #23892, #6447, #14979, #1128, #12513, #32595, #29179, #3602, #21057, #3221, #939, #8914, #20489, #21245, #6058, #6820 ) ),
 .UNSPECIFIED., .F., .F., .F. ) 
 B_SPLINE_SURFACE_WITH_KNOTS ( ( 2, 2 ),
 ( 3, 2, 2, 2, 2, 2, 2, 2, 2, 2, 2, 2, 2, 2, 2, 2, 2, 2, 2, 2, 2, 2, 2, 2, 2, 2, 2, 2, 2, 2, 2, 2, 2, 2, 2, 2, 2, 2, 2, 2, 2, 2, 2, 2, 2, 2, 2, 2, 2, 2, 2, 2, 2, 2, 2, 2, 2, 2, 2, 2, 2, 2, 2, 2, 2, 2, 2, 3 ),
 ( 0.000000000000000000, 1.000000000000000000 ),
 ( 0.000000000000000000, 0.01388888888888888812, 0.02777777777777777624, 0.04166666666666666435, 0.05555555555555555247, 0.06944444444444444753, 0.08333333333333332871, 0.09722222222222222376, 0.1111111111111111049, 0.1250000000000000000, 0.1388888888888888951, 0.1527777777777777901, 0.1666666666666666574, 0.1805555555555555525, 0.1944444444444444475, 0.2083333333333333426, 0.2222222222222222099, 0.2361111111111111049, 0.2500000000000000000, 0.2638888888888888951, 0.2777777777777777901, 0.2916666666666666852, 0.3055555555555555802, 0.3194444444444444198, 0.3333333333333333148, 0.3472222222222222099, 0.3611111111111111049, 0.3750000000000000000, 0.3888888888888888951, 0.4027777777777777901, 0.4166666666666666852, 0.4305555555555555802, 0.4444444444444444198, 0.4583333333333333148, 0.4722222222222222099, 0.4861111111111111049, 0.5000000000000000000, 0.5138888888888888395, 0.5277777777777777901, 0.5416666666666666297, 0.5555555555555555802, 0.5694444444444444198, 0.5833333333333333703, 0.5972222222222222099, 0.6111111111111111605, 0.6250000000000000000, 0.6388888888888888395, 0.6527777777777777901, 0.6666666666666666297, 0.6805555555555555802, 0.6944444444444444198, 0.7083333333333333703, 0.7222222222222222099, 0.7361111111111111605, 0.7500000000000000000, 0.7638888888888888395, 0.7777777777777777901, 0.7916666666666666297, 0.8055555555555555802, 0.8194444444444444198, 0.8333333333333333703, 0.8472222222222222099, 0.8611111111111111605, 0.8750000000000000000, 0.8888888888888888395, 0.9027777777777777901, 0.9166666666666666297, 0.9258785558164617235 ),
 .UNSPECIFIED. ) 
 GEOMETRIC_REPRESENTATION_ITEM ( )  RATIONAL_B_SPLINE_SURFACE ( (
 ( 1.000000000000000000, 0.8660254037844387076, 1.000000000000000000, 0.8660254037844387076, 1.000000000000000000, 0.8660254037844387076, 1.000000000000000000, 0.8660254037844387076, 1.000000000000000000, 0.8660254037844387076, 1.000000000000000000, 0.8660254037844387076, 1.000000000000000000, 0.8660254037844387076, 1.000000000000000000, 0.8660254037844387076, 1.000000000000000000, 0.8660254037844387076, 1.000000000000000000, 0.8660254037844387076, 1.000000000000000000, 0.8660254037844387076, 1.000000000000000000, 0.8660254037844387076, 1.000000000000000000, 0.8660254037844387076, 1.000000000000000000, 0.8660254037844387076, 1.000000000000000000, 0.8660254037844387076, 1.000000000000000000, 0.8660254037844387076, 1.000000000000000000, 0.8660254037844387076, 1.000000000000000000, 0.8660254037844387076, 1.000000000000000000, 0.8660254037844387076, 1.000000000000000000, 0.8660254037844387076, 1.000000000000000000, 0.8660254037844387076, 1.000000000000000000, 0.8660254037844387076, 1.000000000000000000, 0.8660254037844387076, 1.000000000000000000, 0.8660254037844387076, 1.000000000000000000, 0.8660254037844387076, 1.000000000000000000, 0.8660254037844387076, 1.000000000000000000, 0.8660254037844387076, 1.000000000000000000, 0.8660254037844387076, 1.000000000000000000, 0.8660254037844387076, 1.000000000000000000, 0.8660254037844387076, 1.000000000000000000, 0.8660254037844387076, 1.000000000000000000, 0.8660254037844387076, 1.000000000000000000, 0.8660254037844387076, 1.000000000000000000, 0.8660254037844387076, 1.000000000000000000, 0.8660254037844387076, 1.000000000000000000, 0.8660254037844387076, 1.000000000000000000, 0.8660254037844387076, 1.000000000000000000, 0.8660254037844387076, 1.000000000000000000, 0.8660254037844387076, 1.000000000000000000, 0.8660254037844387076, 1.000000000000000000, 0.8660254037844387076, 1.000000000000000000, 0.8660254037844387076, 1.000000000000000000, 0.8660254037844387076, 1.000000000000000000, 0.8660254037844387076, 1.000000000000000000, 0.8660254037844387076, 1.000000000000000000, 0.8660254037844387076, 1.000000000000000000, 0.8660254037844387076, 1.000000000000000000, 0.8660254037844387076, 1.000000000000000000, 0.8660254037844387076, 1.000000000000000000, 0.8660254037844387076, 1.000000000000000000, 0.8660254037844387076, 1.000000000000000000, 0.8660254037844387076, 1.000000000000000000, 0.8660254037844387076, 1.000000000000000000, 0.8660254037844387076, 1.000000000000000000, 0.8660254037844387076, 1.000000000000000000, 0.8660254037844387076, 1.000000000000000000, 0.8660254037844387076, 1.000000000000000000, 0.8660254037844387076, 1.000000000000000000, 0.8660254037844387076, 1.000000000000000000, 0.8660254037844387076, 1.000000000000000000, 0.8660254037844387076, 1.000000000000000000, 0.8660254037844387076, 1.000000000000000000, 0.8660254037844387076, 1.000000000000000000, 0.8660254037844387076, 1.000000000000000000, 0.8660254037844387076, 1.000000000000000000, 0.8660254037844387076, 1.000000000000000000, 0.9111405426957062126, 0.9401542251575389919),
 ( 1.000000000000000000, 0.8660254037844387076, 1.000000000000000000, 0.8660254037844387076, 1.000000000000000000, 0.8660254037844387076, 1.000000000000000000, 0.8660254037844387076, 1.000000000000000000, 0.8660254037844387076, 1.000000000000000000, 0.8660254037844387076, 1.000000000000000000, 0.8660254037844387076, 1.000000000000000000, 0.8660254037844387076, 1.000000000000000000, 0.8660254037844387076, 1.000000000000000000, 0.8660254037844387076, 1.000000000000000000, 0.8660254037844387076, 1.000000000000000000, 0.8660254037844387076, 1.000000000000000000, 0.8660254037844387076, 1.000000000000000000, 0.8660254037844387076, 1.000000000000000000, 0.8660254037844387076, 1.000000000000000000, 0.8660254037844387076, 1.000000000000000000, 0.8660254037844387076, 1.000000000000000000, 0.8660254037844387076, 1.000000000000000000, 0.8660254037844387076, 1.000000000000000000, 0.8660254037844387076, 1.000000000000000000, 0.8660254037844387076, 1.000000000000000000, 0.8660254037844387076, 1.000000000000000000, 0.8660254037844387076, 1.000000000000000000, 0.8660254037844387076, 1.000000000000000000, 0.8660254037844387076, 1.000000000000000000, 0.8660254037844387076, 1.000000000000000000, 0.8660254037844387076, 1.000000000000000000, 0.8660254037844387076, 1.000000000000000000, 0.8660254037844387076, 1.000000000000000000, 0.8660254037844387076, 1.000000000000000000, 0.8660254037844387076, 1.000000000000000000, 0.8660254037844387076, 1.000000000000000000, 0.8660254037844387076, 1.000000000000000000, 0.8660254037844387076, 1.000000000000000000, 0.8660254037844387076, 1.000000000000000000, 0.8660254037844387076, 1.000000000000000000, 0.8660254037844387076, 1.000000000000000000, 0.8660254037844387076, 1.000000000000000000, 0.8660254037844387076, 1.000000000000000000, 0.8660254037844387076, 1.000000000000000000, 0.8660254037844387076, 1.000000000000000000, 0.8660254037844387076, 1.000000000000000000, 0.8660254037844387076, 1.000000000000000000, 0.8660254037844387076, 1.000000000000000000, 0.8660254037844387076, 1.000000000000000000, 0.8660254037844387076, 1.000000000000000000, 0.8660254037844387076, 1.000000000000000000, 0.8660254037844387076, 1.000000000000000000, 0.8660254037844387076, 1.000000000000000000, 0.8660254037844387076, 1.000000000000000000, 0.8660254037844387076, 1.000000000000000000, 0.8660254037844387076, 1.000000000000000000, 0.8660254037844387076, 1.000000000000000000, 0.8660254037844387076, 1.000000000000000000, 0.8660254037844387076, 1.000000000000000000, 0.8660254037844387076, 1.000000000000000000, 0.8660254037844387076, 1.000000000000000000, 0.8660254037844387076, 1.000000000000000000, 0.8660254037844387076, 1.000000000000000000, 0.8660254037844387076, 1.000000000000000000, 0.8660254037844387076, 1.000000000000000000, 0.8660254037844387076, 1.000000000000000000, 0.8660254037844387076, 1.000000000000000000, 0.8660254037844387076, 1.000000000000000000, 0.8660254037844387076, 1.000000000000000000, 0.8660254037844387076, 1.000000000000000000, 0.9111405426957062126, 0.9401542251575389919) ) ) 
 REPRESENTATION_ITEM ( '' )  SURFACE ( )  );
#18828=CARTESIAN_POINT ( 'NONE',  ( 27.24356964375000700, 197.7406250006145285, 15.72908226750537075 ) ) ;
#18833=( BOUNDED_CURVE ( )  B_SPLINE_CURVE ( 2, ( #3335, #4090, #1050, #21168, #27213, #6948, #672, #35170, #12243 ),
 .UNSPECIFIED., .F., .F. ) 
 B_SPLINE_CURVE_WITH_KNOTS ( ( 3, 2, 2, 2, 3 ),
 ( 0.2291666666666666574, 0.2361111111111111049, 0.2500000000000000000, 0.2638888888888888951, 0.2708333333333333703 ),
 .UNSPECIFIED. ) 
 CURVE ( )  GEOMETRIC_REPRESENTATION_ITEM ( )  RATIONAL_B_SPLINE_CURVE ( ( 0.9330127018922194093, 0.9330127018922194093, 1.000000000000000000, 0.8660254037844387076, 1.000000000000000000, 0.8660254037844387076, 1.000000000000000000, 0.9330127018922190762, 0.9330127018922194093 ) ) 
 REPRESENTATION_ITEM ( '' )  );
#18865=CARTESIAN_POINT ( 'NONE',  ( 13.62178482187499640, 198.3031250006145285, -23.59362340125807123 ) ) ;
#18874=EDGE_LOOP ( 'NONE', ( #8951, #16217, #28875, #32072, #27196, #6228, #3794, #23763, #20153, #4957, #24023, #32419, #8418, #35456, #18691, #1476, #26913, #26311, #18703, #5792, #34146, #2327, #3243, #19632, #6511, #16960 ) ) ;
#18880=CARTESIAN_POINT ( 'NONE',  ( 13.49999999999999645, 196.7000000000000171, -23.38268590217984766 ) ) ;
#18897=SURFACE_STYLE_USAGE ( .BOTH. , #16232 ) ;
#18909=ORIENTED_EDGE ( 'NONE', *, *, #19711, .F. ) ;
#18910=CARTESIAN_POINT ( 'NONE',  ( -26.99999999999999645, 196.1000000012290627, 15.58845726811991561 ) ) ;
#18939=EDGE_CURVE ( 'NONE', #11516, #1318, #28628, .T. ) ;
#18956=CARTESIAN_POINT ( 'NONE',  ( -27.00000000000000355, 197.7125000000000057, -15.58845726811989429 ) ) ;
#18984=( BOUNDED_CURVE ( )  B_SPLINE_CURVE ( 2, ( #6913, #15627, #19046, #24347, #27557, #1396, #35889, #4056, #24157 ),
 .UNSPECIFIED., .F., .F. ) 
 B_SPLINE_CURVE_WITH_KNOTS ( ( 3, 2, 2, 2, 3 ),
 ( 0.3125000000000000000, 0.3194444444444444198, 0.3333333333333333148, 0.3472222222222222099, 0.3541666666666666852 ),
 .UNSPECIFIED. ) 
 CURVE ( )  GEOMETRIC_REPRESENTATION_ITEM ( )  RATIONAL_B_SPLINE_CURVE ( ( 0.9330127018922194093, 0.9330127018922194093, 1.000000000000000000, 0.8660254037844387076, 1.000000000000000000, 0.8660254037844387076, 1.000000000000000000, 0.9330127018922190762, 0.9330127018922194093 ) ) 
 REPRESENTATION_ITEM ( '' )  );
#18986=CARTESIAN_POINT ( 'NONE',  ( 13.62178482187501416, 196.8031250006145285, 23.59362340125806767 ) ) ;
#19002=DIRECTION ( 'NONE',  ( 1.000000000000000000, 0.000000000000000000, 0.000000000000000000 ) ) ;
#19005=ORIENTED_EDGE ( 'NONE', *, *, #19096, .T. ) ;
#19011=CARTESIAN_POINT ( 'NONE',  ( 27.24356964375000700, 197.2906250006145399, 15.72908226750537075 ) ) ;
#19046=CARTESIAN_POINT ( 'NONE',  ( -13.49999999999998401, 198.2750000000000057, 23.38268590217985476 ) ) ;
#19052=VERTEX_POINT ( 'NONE', #30512 ) ;
#19054=CARTESIAN_POINT ( 'NONE',  ( -1.926257025242585782E-15, 196.9906250006145001, -31.45816453501076637 ) ) ;
#19055=CARTESIAN_POINT ( 'NONE',  ( 5.778771075727756162E-15, 199.5218750006145854, 31.45816453501075927 ) ) ;
#19056=CARTESIAN_POINT ( 'NONE',  ( 1.120210788295102201E-13, 195.8375000000000057, -27.00000000000000711 ) ) ;
#19068=CARTESIAN_POINT ( 'NONE',  ( 5.727106289114498080E-15, 197.4124999999999943, 31.17691453623979214 ) ) ;
#19076=CARTESIAN_POINT ( 'NONE',  ( -13.49999999999998401, 196.4750000000000227, 23.38268590217985476 ) ) ;
#19083=( LENGTH_UNIT ( ) NAMED_UNIT ( * ) SI_UNIT ( .MILLI., .METRE. ) );
#19096=EDGE_CURVE ( 'NONE', #3136, #26034, #4532, .T. ) ;
#19114=ORIENTED_EDGE ( 'NONE', *, *, #29804, .T. ) ;
#19142=CARTESIAN_POINT ( 'NONE',  ( 27.00000000000001421, 196.1375000000000171, 15.58845726811988897 ) ) ;
#19158=EDGE_CURVE ( 'NONE', #28452, #21721, #33068, .T. ) ;
#19164=CARTESIAN_POINT ( 'NONE',  ( -27.24356964374999279, 195.3968750006145285, 15.72908226750539384 ) ) ;
#19168=AXIS2_PLACEMENT_3D ( 'NONE', #4573, #1540, #16149 ) ;
#19176=CARTESIAN_POINT ( 'NONE',  ( -13.50000000000000533, 198.2375000012290229, -23.38268590217984411 ) ) ;
#19197=CARTESIAN_POINT ( 'NONE',  ( 0.000000000000000000, 200.0000000000000000, -27.00000000000000355 ) ) ;
#19201=CARTESIAN_POINT ( 'NONE',  ( -13.62178482187498396, 197.1781250006145569, 23.59362340125808188 ) ) ;
#19217=ORIENTED_EDGE ( 'NONE', *, *, #13142, .T. ) ;
#19220=AXIS2_PLACEMENT_3D ( 'NONE', #36119, #2686, #28834 ) ;
#19221=CARTESIAN_POINT ( 'NONE',  ( 3.253724281355069334E-15, 199.8875000000000455, -27.00000000000000000 ) ) ;
#19229=CARTESIAN_POINT ( 'NONE',  ( 1.069080835302379631E-14, 197.9750000012290343, 27.00000000000000000 ) ) ;
#19243=CARTESIAN_POINT ( 'NONE',  ( 27.24356964374999279, 196.0156250006145342, -15.72908226750539207 ) ) ;
#19244=CARTESIAN_POINT ( 'NONE',  ( -27.24356964375000345, 197.6093750006145342, 0.000000000000000000 ) ) ;
#19247=CARTESIAN_POINT ( 'NONE',  ( 7.234628195640322446, 195.6325961894323484, 26.99999999999999645 ) ) ;
#19260=CARTESIAN_POINT ( 'NONE',  ( 26.99999999999999645, 197.5624999999999716, -15.58845726811990495 ) ) ;
#19268=LINE ( 'NONE', #7501, #37163 ) ;
#19321=EDGE_CURVE ( 'NONE', #32085, #16548, #19520, .T. ) ;
#19354=CARTESIAN_POINT ( 'NONE',  ( 27.24356964375000700, 195.5468750006145342, 15.72908226750537075 ) ) ;
#19366=CARTESIAN_POINT ( 'NONE',  ( -13.49999999999998401, 197.9375000012290400, 23.38268590217985476 ) ) ;
#19385=ORIENTED_EDGE ( 'NONE', *, *, #27451, .T. ) ;
#19389=CARTESIAN_POINT ( 'NONE',  ( -13.62178482187500528, 195.2281250006145399, -23.59362340125807123 ) ) ;
#19421=ORIENTED_EDGE ( 'NONE', *, *, #12862, .T. ) ;
#19423=CARTESIAN_POINT ( 'NONE',  ( -27.24356964375000345, 195.3031250006145285, 0.000000000000000000 ) ) ;
#19424=CARTESIAN_POINT ( 'NONE',  ( 13.62178482187501416, 199.1093750006145342, 23.59362340125806767 ) ) ;
#19441=CARTESIAN_POINT ( 'NONE',  ( 13.50000000000001421, 196.5500000000000114, 23.38268590217984055 ) ) ;
#19520=LINE ( 'NONE', #27472, #6669 ) ;
#19536=ORIENTED_EDGE ( 'NONE', *, *, #7794, .T. ) ;
#19547=CARTESIAN_POINT ( 'NONE',  ( 13.49999999999999645, 199.0625000012290400, -23.38268590217984766 ) ) ;
#19552=CARTESIAN_POINT ( 'NONE',  ( 0.000000000000000000, 200.0000000000000000, -27.00000000000000355 ) ) ;
#19568=CARTESIAN_POINT ( 'NONE',  ( 27.24356964374999635, 196.9156250006145399, -15.72908226750539029 ) ) ;
#19569=DIRECTION ( 'NONE',  ( 0.000000000000000000, -1.000000000000000000, 0.000000000000000000 ) ) ;
#19573=EDGE_CURVE ( 'NONE', #4926, #10170, #16145, .T. ) ;
#19583=EDGE_CURVE ( 'NONE', #32564, #15189, #26749, .T. ) ;
#19596=ORIENTED_EDGE ( 'NONE', *, *, #15622, .F. ) ;
#19609=CARTESIAN_POINT ( 'NONE',  ( 13.62178482187499640, 195.1531250006145513, -23.59362340125807123 ) ) ;
#19611=CARTESIAN_POINT ( 'NONE',  ( -13.62178482187498396, 198.1343750006145399, 23.59362340125808188 ) ) ;
#19629=CARTESIAN_POINT ( 'NONE',  ( 13.50000000000001421, 195.2000000000000171, 23.38268590217984055 ) ) ;
#19632=ORIENTED_EDGE ( 'NONE', *, *, #25391, .F. ) ;
#19645=DIRECTION ( 'NONE',  ( 1.000000000000000000, 0.000000000000000000, 0.000000000000000000 ) ) ;
#19708=CARTESIAN_POINT ( 'NONE',  ( -27.00000000000000355, 194.7125000012290172, 0.000000000000000000 ) ) ;
#19711=EDGE_CURVE ( 'NONE', #36421, #8730, #11262, .T. ) ;
#19738=CARTESIAN_POINT ( 'NONE',  ( -27.00000000000000355, 199.6250000012290684, -15.58845726811989429 ) ) ;
#19761=CARTESIAN_POINT ( 'NONE',  ( 13.62178482187501416, 195.4531250006145342, 23.59362340125806767 ) ) ;
#19775=AXIS2_PLACEMENT_3D ( 'NONE', #4945, #16158, #27707 ) ;
#19799=CARTESIAN_POINT ( 'NONE',  ( 27.24356964374999635, 198.7718750006145569, -15.72908226750539029 ) ) ;
#19803=EDGE_CURVE ( 'NONE', #4030, #20323, #30645, .T. ) ;
#19810=CARTESIAN_POINT ( 'NONE',  ( -1.045839947578415010E-13, 196.0625000000000284, 27.00000000000000355 ) ) ;
#19816=CARTESIAN_POINT ( 'NONE',  ( 27.24356964375000345, 199.6343750006145399, -3.336375036156643733E-15 ) ) ;
#19818=ORIENTED_EDGE ( 'NONE', *, *, #6200, .F. ) ;
#19858=DIRECTION ( 'NONE',  ( -0.000000000000000000, -1.000000000000000000, -0.000000000000000000 ) ) ;
#19890=CARTESIAN_POINT ( 'NONE',  ( -4.694659320240884604E-14, 197.0750000012290570, 27.00000000000000000 ) ) ;
#19917=CARTESIAN_POINT ( 'NONE',  ( -13.50000000000000533, 198.6875000012290400, -23.38268590217984411 ) ) ;
#19941=CARTESIAN_POINT ( 'NONE',  ( -20.86978560514296532, 194.8213513911397570, -17.51182845191284798 ) ) ;
#19974=CARTESIAN_POINT ( 'NONE',  ( 27.24356964375000345, 195.5281250006145228, -3.336375036156643733E-15 ) ) ;
#19976=CARTESIAN_POINT ( 'NONE',  ( -27.24356964375000345, 199.8031250006145285, 0.000000000000000000 ) ) ;
#19984=ORIENTED_EDGE ( 'NONE', *, *, #23790, .F. ) ;
#19992=CARTESIAN_POINT ( 'NONE',  ( -13.62178482187500528, 199.3343750006145569, -23.59362340125807123 ) ) ;
#20064=CARTESIAN_POINT ( 'NONE',  ( 0.000000000000000000, 200.0000000000000000, 0.000000000000000000 ) ) ;
#20068=CARTESIAN_POINT ( 'NONE',  ( -27.00000000000000355, 196.9625000012290172, 0.000000000000000000 ) ) ;
#20094=CARTESIAN_POINT ( 'NONE',  ( -1.909035429704832693E-15, 197.3000000012290513, -31.17691453623979214 ) ) ;
#20111=ORIENTED_EDGE ( 'NONE', *, *, #18939, .T. ) ;
#20122=CARTESIAN_POINT ( 'NONE',  ( -27.24356964375000345, 199.8593750006145342, 0.000000000000000000 ) ) ;
#20134=CARTESIAN_POINT ( 'NONE',  ( 13.62178482187499640, 199.2031250006145342, -23.59362340125807123 ) ) ;
#20144=EDGE_LOOP ( 'NONE', ( #15203, #22278, #34251, #4538 ) ) ;
#20153=ORIENTED_EDGE ( 'NONE', *, *, #26807, .F. ) ;
#20154=CARTESIAN_POINT ( 'NONE',  ( -27.00000000000000355, 198.7625000012290286, 0.000000000000000000 ) ) ;
#20155=CARTESIAN_POINT ( 'NONE',  ( 13.62178482187501416, 196.4093750006145456, 23.59362340125806767 ) ) ;
#20175=CARTESIAN_POINT ( 'NONE',  ( 13.62178482187501416, 199.1093750006145342, 23.59362340125806767 ) ) ;
#20197=CARTESIAN_POINT ( 'NONE',  ( -3.253724281355068545E-15, 196.2874999999999659, -27.00000000000000355 ) ) ;
#20210=CARTESIAN_POINT ( 'NONE',  ( -3.253724281355068545E-15, 197.3000000012290229, -27.00000000000000355 ) ) ;
#20223=VECTOR ( 'NONE', #18739, 1000.000000000000000 ) ;
#20272=EDGE_CURVE ( 'NONE', #25162, #5600, #16718, .T. ) ;
#20283=CARTESIAN_POINT ( 'NONE',  ( -13.49999999999998401, 196.5875000012290457, 23.38268590217985476 ) ) ;
#20308=CARTESIAN_POINT ( 'NONE',  ( -27.24356964374999635, 194.8906250006145342, 15.72908226750539384 ) ) ;
#20323=VERTEX_POINT ( 'NONE', #6 ) ;
#20348=CARTESIAN_POINT ( 'NONE',  ( 27.24356964374999635, 196.5218750006145569, -15.72908226750539029 ) ) ;
#20352=AXIS2_PLACEMENT_3D ( 'NONE', #14796, #26158, #17648 ) ;
#20358=CARTESIAN_POINT ( 'NONE',  ( 27.00000000000000355, 197.1875000012290400, -3.306546357697854128E-15 ) ) ;
#20366=CARTESIAN_POINT ( 'NONE',  ( -13.62178482187498396, 199.4843750006145626, 23.59362340125808188 ) ) ;
#20395=CARTESIAN_POINT ( 'NONE',  ( 13.62178482187499640, 199.6531250006145228, -23.59362340125807123 ) ) ;
#20418=FACE_OUTER_BOUND ( 'NONE', #30267, .T. ) ;
#20471=CARTESIAN_POINT ( 'NONE',  ( -26.99999999999998934, 196.5500000012290229, 15.58845726811991561 ) ) ;
#20482=VECTOR ( 'NONE', #13269, 1000.000000000000000 ) ;
#20489=CARTESIAN_POINT ( 'NONE',  ( -27.24356964374999635, 194.9468750006145399, 15.72908226750539384 ) ) ;
#20502=CARTESIAN_POINT ( 'NONE',  ( 5.778771075727756162E-15, 199.5218750006145569, 31.45816453501076637 ) ) ;
#20503=VECTOR ( 'NONE', #29840, 1000.000000000000000 ) ;
#20515=CARTESIAN_POINT ( 'NONE',  ( -1.926257025242585782E-15, 198.7906250006145399, -31.45816453501075927 ) ) ;
#20534=CARTESIAN_POINT ( 'NONE',  ( -27.24356964374999990, 196.6718750006145342, -15.72908226750537786 ) ) ;
#20550=CARTESIAN_POINT ( 'NONE',  ( 13.62178482187499640, 198.3593750006145342, -23.59362340125807123 ) ) ;
#20551=ORIENTED_EDGE ( 'NONE', *, *, #18504, .F. ) ;
#20555=CARTESIAN_POINT ( 'NONE',  ( -7.234628195640263826, 195.4075961894323825, -27.00000000000003553 ) ) ;
#20574=DIRECTION ( 'NONE',  ( -0.000000000000000000, -1.000000000000000000, -0.000000000000000000 ) ) ;
#20577=CARTESIAN_POINT ( 'NONE',  ( 5.778771075727756162E-15, 199.0156250006145342, 31.45816453501076637 ) ) ;
#20591=EDGE_CURVE ( 'NONE', #5529, #21803, #21680, .T. ) ;
#20647=EDGE_LOOP ( 'NONE', ( #32941, #33178, #33882, #14319 ) ) ;
#20655=CARTESIAN_POINT ( 'NONE',  ( -13.50000000000000533, 195.5375000012290343, -23.38268590217984411 ) ) ;
#20672=CARTESIAN_POINT ( 'NONE',  ( 27.24356964375000700, 195.9968750006145513, 15.72908226750537075 ) ) ;
#20678=CARTESIAN_POINT ( 'NONE',  ( 0.000000000000000000, 200.0000000000000000, 0.000000000000000000 ) ) ;
#20683=CARTESIAN_POINT ( 'NONE',  ( 27.00000000000001421, 198.3875000000000171, 15.58845726811988897 ) ) ;
#20696=CARTESIAN_POINT ( 'NONE',  ( -13.62178482187498396, 198.0781250006145342, 23.59362340125808188 ) ) ;
#20718=CARTESIAN_POINT ( 'NONE',  ( -13.62178482187500528, 195.2843750006145456, -23.59362340125807123 ) ) ;
#20725=CARTESIAN_POINT ( 'NONE',  ( 3.306546357697854128E-15, 200.0000000000000000, 27.00000000000000355 ) ) ;
#20735=CARTESIAN_POINT ( 'NONE',  ( 13.62178482187501416, 198.2093750006145285, 23.59362340125806767 ) ) ;
#20758=PLANE ( 'NONE',  #18044 ) ;
#20761=CARTESIAN_POINT ( 'NONE',  ( 3.306546357697854128E-15, 200.0000000000000000, 27.00000000000000355 ) ) ;
#20765=EDGE_CURVE ( 'NONE', #55, #32329, #8602, .T. ) ;
#20787=CARTESIAN_POINT ( 'NONE',  ( 0.000000000000000000, 200.0000000000000000, -25.00000000000000000 ) ) ;
#20798=CYLINDRICAL_SURFACE ( 'NONE', #9486, 27.00000000000000355 ) ;
#20821=CIRCLE ( 'NONE', #4465, 25.00000000000000000 ) ;
#20846=CARTESIAN_POINT ( 'NONE',  ( 27.00000000000001066, 195.8000000012290513, 15.58845726811988897 ) ) ;
#20868=CARTESIAN_POINT ( 'NONE',  ( 27.24356964374999635, 196.5218750006145569, -15.72908226750539029 ) ) ;
#20877=CARTESIAN_POINT ( 'NONE',  ( 27.00000000000000355, 198.8750000000000284, -3.306546357697854128E-15 ) ) ;
#20879=CARTESIAN_POINT ( 'NONE',  ( 27.24356964374999279, 198.7718750006145569, -15.72908226750539207 ) ) ;
#20888=CARTESIAN_POINT ( 'NONE',  ( -13.62178482187500528, 199.7281250006145399, -23.59362340125807123 ) ) ;
#20894=VECTOR ( 'NONE', #3653, 1000.000000000000000 ) ;
#20907=EDGE_CURVE ( 'NONE', #32162, #5775, #37107, .T. ) ;
#20913=CARTESIAN_POINT ( 'NONE',  ( 13.62178482187499640, 197.8531250006145399, -23.59362340125807123 ) ) ;
#20928=CARTESIAN_POINT ( 'NONE',  ( 27.24356964375000345, 197.8343750006145569, -3.336375036156643733E-15 ) ) ;
#20959=CARTESIAN_POINT ( 'NONE',  ( -1.045839947578415010E-13, 194.8250000012290570, 27.00000000000000355 ) ) ;
#20972=VECTOR ( 'NONE', #33980, 1000.000000000000000 ) ;
#20976=EDGE_CURVE ( 'NONE', #33186, #19052, #25317, .T. ) ;
#21036=CARTESIAN_POINT ( 'NONE',  ( -13.49999999999998401, 194.7875000012290343, 23.38268590217985476 ) ) ;
#21057=CARTESIAN_POINT ( 'NONE',  ( 27.24356964375000700, 195.0968750006145456, 15.72908226750537075 ) ) ;
#21069=CARTESIAN_POINT ( 'NONE',  ( 13.62178482187501416, 197.7593750006145399, 23.59362340125806767 ) ) ;
#21079=CARTESIAN_POINT ( 'NONE',  ( -7.234628195640313564, 199.5700961906613884, -27.00000000000000355 ) ) ;
#21083=CARTESIAN_POINT ( 'NONE',  ( 13.62178482187499640, 197.4031250006145228, -23.59362340125807123 ) ) ;
#21105=CARTESIAN_POINT ( 'NONE',  ( 27.24356964375000345, 197.7781250006145228, -3.336375036156643733E-15 ) ) ;
#21106=CARTESIAN_POINT ( 'NONE',  ( 27.00000000000001421, 198.0500000012290513, 15.58845726811988897 ) ) ;
#21119=CARTESIAN_POINT ( 'NONE',  ( -27.24356964375000345, 197.6093750006145342, 0.000000000000000000 ) ) ;
#21144=CARTESIAN_POINT ( 'NONE',  ( -27.24356964375000345, 198.4531250006145342, 0.000000000000000000 ) ) ;
#21161=CARTESIAN_POINT ( 'NONE',  ( -13.49999999999998401, 199.1750000000000114, 23.38268590217985476 ) ) ;
#21167=CARTESIAN_POINT ( 'NONE',  ( 1.069080835302379631E-14, 196.6250000012290400, 27.00000000000000000 ) ) ;
#21168=CARTESIAN_POINT ( 'NONE',  ( -26.99999999999999645, 198.3500000012290343, 15.58845726811991561 ) ) ;
#21202=CARTESIAN_POINT ( 'NONE',  ( 7.234628195640312676, 199.8674038105676800, -27.00000000000000711 ) ) ;
#21224=CARTESIAN_POINT ( 'NONE',  ( 13.50000000000001421, 194.8625000012290513, 23.38268590217984055 ) ) ;
#21245=CARTESIAN_POINT ( 'NONE',  ( -27.24356964375000345, 194.9093750006145456, 0.000000000000000000 ) ) ;
#21255=CARTESIAN_POINT ( 'NONE',  ( 26.99999999999999645, 199.4750000012290343, -15.58845726811990495 ) ) ;
#21257=CARTESIAN_POINT ( 'NONE',  ( -27.24356964374999279, 198.0968750006145456, 15.72908226750539384 ) ) ;
#21269=CARTESIAN_POINT ( 'NONE',  ( -1.926257025242585782E-15, 195.6406250006145058, -31.45816453501075927 ) ) ;
#21294=CARTESIAN_POINT ( 'NONE',  ( 13.62178482187499640, 198.3031250006145285, -23.59362340125807123 ) ) ;
#21295=CARTESIAN_POINT ( 'NONE',  ( -1.045839947578415010E-13, 196.5125000000000455, 27.00000000000000355 ) ) ;
#21334=CARTESIAN_POINT ( 'NONE',  ( 13.62178482187501416, 197.2531250006145456, 23.59362340125806767 ) ) ;
#21335=CARTESIAN_POINT ( 'NONE',  ( -1.926257025242585782E-15, 199.7468750006145513, -31.45816453501075927 ) ) ;
#21349=CARTESIAN_POINT ( 'NONE',  ( -1.909035429704832693E-15, 199.4375000000000284, -31.17691453623979214 ) ) ;
#21352=ORIENTED_EDGE ( 'NONE', *, *, #5298, .F. ) ;
#21356=CARTESIAN_POINT ( 'NONE',  ( 0.000000000000000000, 200.0000000000000000, 0.000000000000000000 ) ) ;
#21410=CARTESIAN_POINT ( 'NONE',  ( -27.00000000000000355, 194.7125000012290172, 0.000000000000000000 ) ) ;
#21421=CARTESIAN_POINT ( 'NONE',  ( 7.234628195640309123, 196.2674038105676573, -27.00000000000000711 ) ) ;
#21428=ADVANCED_FACE ( 'NONE', ( #10269 ), #34134, .T. ) ;
#21440=CARTESIAN_POINT ( 'NONE',  ( 7.234628195640337545, 198.5174038105677141, -26.99999999999999289 ) ) ;
#21442=CARTESIAN_POINT ( 'NONE',  ( 13.62178482187499640, 198.3593750006145342, -23.59362340125807123 ) ) ;
#21457=CARTESIAN_POINT ( 'NONE',  ( 27.24356964375000345, 195.5281250006145228, -3.336375036156643733E-15 ) ) ;
#21471=CIRCLE ( 'NONE', #25069, 27.00000000000000355 ) ;
#21483=CARTESIAN_POINT ( 'NONE',  ( -27.24356964374999635, 199.3906250006145342, 15.72908226750539384 ) ) ;
#21488=EDGE_CURVE ( 'NONE', #36971, #1101, #1548, .T. ) ;
#21491=ORIENTED_EDGE ( 'NONE', *, *, #31566, .T. ) ;
#21520=CARTESIAN_POINT ( 'NONE',  ( 27.24356964375000345, 197.3281250006145342, -3.336375036156643733E-15 ) ) ;
#21521=CARTESIAN_POINT ( 'NONE',  ( 27.24356964375000700, 199.5968750006145456, 15.72908226750537075 ) ) ;
#21537=CARTESIAN_POINT ( 'NONE',  ( 13.49999999999999645, 197.1500000000000057, -23.38268590217984766 ) ) ;
#21540=ORIENTED_EDGE ( 'NONE', *, *, #3211, .T. ) ;
#21586=CARTESIAN_POINT ( 'NONE',  ( 0.000000000000000000, 200.0000000000000000, 0.000000000000000000 ) ) ;
#21622=CARTESIAN_POINT ( 'NONE',  ( 13.50000000000001421, 199.3625000012290513, 23.38268590217984055 ) ) ;
#21626=CARTESIAN_POINT ( 'NONE',  ( 5.778771075727756162E-15, 196.8218750006145683, 31.45816453501076637 ) ) ;
#21637=CARTESIAN_POINT ( 'NONE',  ( -27.24356964374999990, 197.0656250006145171, -15.72908226750537786 ) ) ;
#21648=CARTESIAN_POINT ( 'NONE',  ( -7.234628195640302017, 195.2549038117967086, 27.00000000000000711 ) ) ;
#21661=CARTESIAN_POINT ( 'NONE',  ( -13.62178482187498396, 198.0781250006145342, 23.59362340125808188 ) ) ;
#21680=( BOUNDED_CURVE ( )  B_SPLINE_CURVE ( 2, ( #20122, #26167, #23335, #5888, #11396, #26540, #17466, #25983, #26352, #20502, #29002, #11579, #11954, #6070, #29191, #3233, #17847, #388, #23712, #23523, #6270, #29385, #31670, #3422, #5699, #570, #12137, #35253, #9307, #20879, #32418, #6462, #2672, #14247, #25796, #22968, #17279, #28820, #14428, #13, #21442, #15747, #12898, #32607, #9493, #24462, #3984, #21257, #36011, #32796, #35445, #12329, #18604, #7221, #21811, #18793, #21069, #30335, #10050, #6646, #6832, #3614, #29956, #24642, #30147, #15939, #29576, #4358, #13087, #24278, #18222, #15370, #23903, #33364, #3793, #15180, #26727, #15558, #7400, #18408, #29762, #21626, #761, #10236, #33177, #26920, #27487, #950, #12525, #1513, #12706, #27115, #24088, #35633, #1138, #35822, #9680, #36192, #9863, #32984, #7037, #4176, #27298, #1329, #10608, #1701, #36566, #28045, #25204, #5106, #22187, #33735, #16124, #22745, #30714, #19354, #34294, #2078, #27675, #19164, #22372, #13273, #16871, #36757, #7776, #25011, #24826, #7590, #10425, #36379, #30894, #4734, #13460, #21999, #31083 ),
 .UNSPECIFIED., .F., .F. ) 
 B_SPLINE_CURVE_WITH_KNOTS ( ( 3, 2, 2, 2, 2, 2, 2, 2, 2, 2, 2, 2, 2, 2, 2, 2, 2, 2, 2, 2, 2, 2, 2, 2, 2, 2, 2, 2, 2, 2, 2, 2, 2, 2, 2, 2, 2, 2, 2, 2, 2, 2, 2, 2, 2, 2, 2, 2, 2, 2, 2, 2, 2, 2, 2, 2, 2, 2, 2, 2, 2, 2, 2, 2, 2, 2, 2, 3 ),
 ( 0.000000000000000000, 0.01388888888888888812, 0.02777777777777777624, 0.04166666666666666435, 0.05555555555555555247, 0.06944444444444444753, 0.08333333333333332871, 0.09722222222222222376, 0.1111111111111111049, 0.1250000000000000000, 0.1388888888888888951, 0.1527777777777777901, 0.1666666666666666574, 0.1805555555555555525, 0.1944444444444444475, 0.2083333333333333426, 0.2222222222222222099, 0.2361111111111111049, 0.2500000000000000000, 0.2638888888888888951, 0.2777777777777777901, 0.2916666666666666852, 0.3055555555555555802, 0.3194444444444444198, 0.3333333333333333148, 0.3472222222222222099, 0.3611111111111111049, 0.3750000000000000000, 0.3888888888888888951, 0.4027777777777777901, 0.4166666666666666852, 0.4305555555555555802, 0.4444444444444444198, 0.4583333333333333148, 0.4722222222222222099, 0.4861111111111111049, 0.5000000000000000000, 0.5138888888888888395, 0.5277777777777777901, 0.5416666666666666297, 0.5555555555555555802, 0.5694444444444444198, 0.5833333333333333703, 0.5972222222222222099, 0.6111111111111111605, 0.6250000000000001110, 0.6388888888888888395, 0.6527777777777777901, 0.6666666666666666297, 0.6805555555555555802, 0.6944444444444444198, 0.7083333333333333703, 0.7222222222222222099, 0.7361111111111111605, 0.7500000000000000000, 0.7638888888888888395, 0.7777777777777777901, 0.7916666666666666297, 0.8055555555555555802, 0.8194444444444444198, 0.8333333333333333703, 0.8472222222222222099, 0.8611111111111111605, 0.8749999999999998890, 0.8888888888888888395, 0.9027777777777777901, 0.9166666666666666297, 0.9258785558164617235 ),
 .UNSPECIFIED. ) 
 CURVE ( )  GEOMETRIC_REPRESENTATION_ITEM ( )  RATIONAL_B_SPLINE_CURVE ( ( 1.000000000000000000, 0.8660254037844387076, 1.000000000000000000, 0.8660254037844387076, 1.000000000000000000, 0.8660254037844387076, 1.000000000000000000, 0.8660254037844387076, 1.000000000000000000, 0.8660254037844387076, 1.000000000000000000, 0.8660254037844387076, 1.000000000000000000, 0.8660254037844387076, 1.000000000000000000, 0.8660254037844387076, 1.000000000000000000, 0.8660254037844387076, 1.000000000000000000, 0.8660254037844387076, 1.000000000000000000, 0.8660254037844387076, 1.000000000000000000, 0.8660254037844387076, 1.000000000000000000, 0.8660254037844387076, 1.000000000000000000, 0.8660254037844387076, 1.000000000000000000, 0.8660254037844387076, 1.000000000000000000, 0.8660254037844387076, 1.000000000000000000, 0.8660254037844387076, 1.000000000000000000, 0.8660254037844387076, 1.000000000000000000, 0.8660254037844387076, 1.000000000000000000, 0.8660254037844387076, 1.000000000000000000, 0.8660254037844387076, 1.000000000000000000, 0.8660254037844387076, 1.000000000000000000, 0.8660254037844387076, 1.000000000000000000, 0.8660254037844387076, 1.000000000000000000, 0.8660254037844387076, 1.000000000000000000, 0.8660254037844387076, 1.000000000000000000, 0.8660254037844387076, 1.000000000000000000, 0.8660254037844387076, 1.000000000000000000, 0.8660254037844387076, 1.000000000000000000, 0.8660254037844387076, 1.000000000000000000, 0.8660254037844387076, 1.000000000000000000, 0.8660254037844387076, 1.000000000000000000, 0.8660254037844387076, 1.000000000000000000, 0.8660254037844387076, 1.000000000000000000, 0.8660254037844387076, 1.000000000000000000, 0.8660254037844387076, 1.000000000000000000, 0.8660254037844387076, 1.000000000000000000, 0.8660254037844387076, 1.000000000000000000, 0.8660254037844387076, 1.000000000000000000, 0.8660254037844387076, 1.000000000000000000, 0.8660254037844387076, 1.000000000000000000, 0.8660254037844387076, 1.000000000000000000, 0.8660254037844387076, 1.000000000000000000, 0.8660254037844387076, 1.000000000000000000, 0.8660254037844387076, 1.000000000000000000, 0.8660254037844387076, 1.000000000000000000, 0.8660254037844387076, 1.000000000000000000, 0.8660254037844387076, 1.000000000000000000, 0.8660254037844387076, 1.000000000000000000, 0.8660254037844387076, 1.000000000000000000, 0.8660254037844387076, 1.000000000000000000, 0.8660254037844387076, 1.000000000000000000, 0.8660254037844387076, 1.000000000000000000, 0.8660254037844387076, 1.000000000000000000, 0.8660254037844387076, 1.000000000000000000, 0.8660254037844387076, 1.000000000000000000, 0.8660254037844387076, 1.000000000000000000, 0.8660254037844387076, 1.000000000000000000, 0.8660254037844387076, 1.000000000000000000, 0.8660254037844387076, 1.000000000000000000, 0.8660254037844387076, 1.000000000000000000, 0.8660254037844387076, 1.000000000000000000, 0.8660254037844387076, 1.000000000000000000, 0.8660254037844387076, 1.000000000000000000, 0.8660254037844387076, 1.000000000000000000, 0.8660254037844387076, 1.000000000000000000, 0.9111405426957062126, 0.9401542251575389919 ) ) 
 REPRESENTATION_ITEM ( '' )  );
#21688=VECTOR ( 'NONE', #20574, 1000.000000000000000 ) ;
#21702=CARTESIAN_POINT ( 'NONE',  ( 27.24356964375000700, 198.1906250006145740, 15.72908226750537075 ) ) ;
#21718=CARTESIAN_POINT ( 'NONE',  ( -27.00000000000000355, 198.6500000000000341, 0.000000000000000000 ) ) ;
#21721=VERTEX_POINT ( 'NONE', #6061 ) ;
#21752=ADVANCED_FACE ( 'NONE', ( #8367 ), #22773, .T. ) ;
#21794=CARTESIAN_POINT ( 'NONE',  ( -4.694659320240884604E-14, 197.8625000000000114, 27.00000000000000000 ) ) ;
#21803=VERTEX_POINT ( 'NONE', #17790 ) ;
#21811=CARTESIAN_POINT ( 'NONE',  ( 27.24356964375000345, 197.8343750006145569, -3.336375036156643733E-15 ) ) ;
#21824=CARTESIAN_POINT ( 'NONE',  ( 13.62178482187501416, 196.3531250006145115, 23.59362340125806767 ) ) ;
#21835=CARTESIAN_POINT ( 'NONE',  ( -26.99999999999999645, 195.2000000012290286, 15.58845726811991561 ) ) ;
#21848=CARTESIAN_POINT ( 'NONE',  ( 13.62178482187501416, 196.8031250006145285, 23.59362340125806767 ) ) ;
#21871=CARTESIAN_POINT ( 'NONE',  ( -13.49999999999998401, 196.9250000000000114, 23.38268590217985476 ) ) ;
#21884=CARTESIAN_POINT ( 'NONE',  ( 5.778771075727756162E-15, 197.2156250006145513, 31.45816453501076637 ) ) ;
#21902=CARTESIAN_POINT ( 'NONE',  ( 13.49999999999999645, 198.5000000000000000, -23.38268590217984766 ) ) ;
#21961=ORIENTED_EDGE ( 'NONE', *, *, #5707, .T. ) ;
#21982=AXIS2_PLACEMENT_3D ( 'NONE', #21356, #32896, #35356 ) ;
#21999=CARTESIAN_POINT ( 'NONE',  ( -27.24356964375000700, 194.8857344423842619, -9.915847606754345733 ) ) ;
#22009=VERTEX_POINT ( 'NONE', #1655 ) ;
#22010=CARTESIAN_POINT ( 'NONE',  ( 5.778771075727756162E-15, 194.9656250006145228, 31.45816453501075927 ) ) ;
#22026=CARTESIAN_POINT ( 'NONE',  ( 7.234628195640295800, 197.8825961894323484, 27.00000000000001066 ) ) ;
#22030=DIRECTION ( 'NONE',  ( -0.000000000000000000, -1.000000000000000000, -0.000000000000000000 ) ) ;
#22035=CARTESIAN_POINT ( 'NONE',  ( 13.62178482187499640, 195.6031250006145115, -23.59362340125807123 ) ) ;
#22059=COLOUR_RGB ( '',0.8941176470588234615, 0.8941176470588234615, 0.8941176470588234615 ) ;
#22073=CARTESIAN_POINT ( 'NONE',  ( -13.62178482187500528, 195.6781250006145569, -23.59362340125807123 ) ) ;
#22074=CARTESIAN_POINT ( 'NONE',  ( 27.24356964375000345, 199.1843750006145228, -3.336375036156643733E-15 ) ) ;
#22091=CARTESIAN_POINT ( 'NONE',  ( -27.00000000000000355, 196.8125000000000000, -15.58845726811989429 ) ) ;
#22120=VECTOR ( 'NONE', #26115, 1000.000000000000000 ) ;
#22173=LINE ( 'NONE', #10967, #4947 ) ;
#22187=CARTESIAN_POINT ( 'NONE',  ( -13.62178482187500528, 195.7343750006145626, -23.59362340125807123 ) ) ;
#22188=ORIENTED_EDGE ( 'NONE', *, *, #22471, .F. ) ;
#22190=( BOUNDED_CURVE ( )  B_SPLINE_CURVE ( 2, ( #11246, #14096, #13915, #2529, #10498, #34183, #25466, #19247, #28121 ),
 .UNSPECIFIED., .F., .F. ) 
 B_SPLINE_CURVE_WITH_KNOTS ( ( 3, 2, 2, 2, 3 ),
 ( 0.7708333333333333703, 0.7777777777777777901, 0.7916666666666666297, 0.8055555555555555802, 0.8125000000000000000 ),
 .UNSPECIFIED. ) 
 CURVE ( )  GEOMETRIC_REPRESENTATION_ITEM ( )  RATIONAL_B_SPLINE_CURVE ( ( 0.9330127018922192983, 0.9330127018922198534, 1.000000000000000000, 0.8660254037844387076, 1.000000000000000000, 0.8660254037844387076, 1.000000000000000000, 0.9330127018922194093, 0.9330127018922194093 ) ) 
 REPRESENTATION_ITEM ( '' )  );
#22192=AXIS2_PLACEMENT_3D ( 'NONE', #8576, #31691, #13900 ) ;
#22200=CARTESIAN_POINT ( 'NONE',  ( 13.49999999999999645, 198.1625000012290343, -23.38268590217984766 ) ) ;
#22221=CARTESIAN_POINT ( 'NONE',  ( 5.778771075727756162E-15, 196.3156250006145171, 31.45816453501075927 ) ) ;
#22224=DIRECTION ( 'NONE',  ( -0.000000000000000000, -1.000000000000000000, -0.000000000000000000 ) ) ;
#22249=CARTESIAN_POINT ( 'NONE',  ( -3.253724281355068545E-15, 195.9500000012290002, -27.00000000000000000 ) ) ;
#22254=DIRECTION ( 'NONE',  ( 0.000000000000000000, -1.000000000000000000, 0.000000000000000000 ) ) ;
#22261=CARTESIAN_POINT ( 'NONE',  ( 27.24356964374999279, 195.5656250006145171, -15.72908226750539207 ) ) ;
#22262=CARTESIAN_POINT ( 'NONE',  ( 27.24356964375000700, 197.3468750006145740, 15.72908226750537075 ) ) ;
#22265=CARTESIAN_POINT ( 'NONE',  ( 7.234628195640269155, 196.1950961906613600, 27.00000000000003197 ) ) ;
#22277=CARTESIAN_POINT ( 'NONE',  ( 27.00000000000001066, 196.5875000000000341, 15.58845726811988897 ) ) ;
#22278=ORIENTED_EDGE ( 'NONE', *, *, #23148, .T. ) ;
#22290=PRESENTATION_STYLE_ASSIGNMENT (( #18897 ) ) ;
#22326=FACE_OUTER_BOUND ( 'NONE', #7391, .T. ) ;
#22344=( BOUNDED_CURVE ( )  B_SPLINE_CURVE ( 2, ( #35269, #29784, #6481, #12349, #18053, #29595, #3632, #15201, #35464 ),
 .UNSPECIFIED., .F., .F. ) 
 B_SPLINE_CURVE_WITH_KNOTS ( ( 3, 2, 2, 2, 3 ),
 ( 0.5208333333333333703, 0.5277777777777777901, 0.5416666666666666297, 0.5555555555555555802, 0.5625000000000000000 ),
 .UNSPECIFIED. ) 
 CURVE ( )  GEOMETRIC_REPRESENTATION_ITEM ( )  RATIONAL_B_SPLINE_CURVE ( ( 0.9330127018922192983, 0.9330127018922198534, 1.000000000000000000, 0.8660254037844387076, 1.000000000000000000, 0.8660254037844387076, 1.000000000000000000, 0.9330127018922194093, 0.9330127018922194093 ) ) 
 REPRESENTATION_ITEM ( '' )  );
#22352=CARTESIAN_POINT ( 'NONE',  ( -26.99999999999999645, 197.7874999999999943, 15.58845726811991561 ) ) ;
#22356=EDGE_CURVE ( 'NONE', #34685, #25286, #35110, .T. ) ;
#22372=CARTESIAN_POINT ( 'NONE',  ( -27.24356964375000345, 195.3593750006145342, 0.000000000000000000 ) ) ;
#22382=CARTESIAN_POINT ( 'NONE',  ( -13.62178482187500528, 195.2281250006145399, -23.59362340125807123 ) ) ;
#22404=( BOUNDED_CURVE ( )  B_SPLINE_CURVE ( 2, ( #23559, #11987, #9722, #17689, #3834, #21106, #26387, #35286, #29613 ),
 .UNSPECIFIED., .F., .F. ) 
 B_SPLINE_CURVE_WITH_KNOTS ( ( 3, 2, 2, 2, 3 ),
 ( 0.2708333333333333703, 0.2777777777777777901, 0.2916666666666666852, 0.3055555555555555802, 0.3125000000000000000 ),
 .UNSPECIFIED. ) 
 CURVE ( )  GEOMETRIC_REPRESENTATION_ITEM ( )  RATIONAL_B_SPLINE_CURVE ( ( 0.9330127018922194093, 0.9330127018922196314, 1.000000000000000000, 0.8660254037844387076, 1.000000000000000000, 0.8660254037844387076, 1.000000000000000000, 0.9330127018922194093, 0.9330127018922194093 ) ) 
 REPRESENTATION_ITEM ( '' )  );
#22406=CARTESIAN_POINT ( 'NONE',  ( -27.24356964375000345, 196.6531250006145513, 0.000000000000000000 ) ) ;
#22444=CARTESIAN_POINT ( 'NONE',  ( 13.62178482187501416, 196.3531250006145115, 23.59362340125806767 ) ) ;
#22445=CARTESIAN_POINT ( 'NONE',  ( -27.24356964374999990, 198.4718750006145171, -15.72908226750537786 ) ) ;
#22461=CARTESIAN_POINT ( 'NONE',  ( 26.99999999999999645, 195.7625000000000171, -15.58845726811990495 ) ) ;
#22471=EDGE_CURVE ( 'NONE', #33186, #25843, #4914, .T. ) ;
#22477=FILL_AREA_STYLE ('',( #10902 ) ) ;
#22541=CARTESIAN_POINT ( 'NONE',  ( 3.253724281355069334E-15, 199.5500000012290513, -27.00000000000000355 ) ) ;
#22566=CARTESIAN_POINT ( 'NONE',  ( 27.24356964374999635, 195.1156250006145001, -15.72908226750539029 ) ) ;
#22593=CARTESIAN_POINT ( 'NONE',  ( 5.778771075727756162E-15, 195.8656250006145285, 31.45816453501075927 ) ) ;
#22597=CARTESIAN_POINT ( 'NONE',  ( 5.438367727407757144E-14, 198.5374999999999943, -27.00000000000000000 ) ) ;
#22633=CARTESIAN_POINT ( 'NONE',  ( -1.926257025242585782E-15, 197.9468750006145399, -31.45816453501075927 ) ) ;
#22636=FACE_BOUND ( 'NONE', #8885, .T. ) ;
#22650=CARTESIAN_POINT ( 'NONE',  ( -26.99999999999998934, 195.0875000000000341, 15.58845726811991561 ) ) ;
#22658=PRODUCT_DEFINITION_FORMATION_WITH_SPECIFIED_SOURCE ( 'ANY', '', #16821, .NOT_KNOWN. ) ;
#22692=CARTESIAN_POINT ( 'NONE',  ( 13.49999999999999645, 197.7125000012290172, -23.38268590217984766 ) ) ;
#22719=LINE ( 'NONE', #25915, #9925 ) ;
#22745=CARTESIAN_POINT ( 'NONE',  ( 27.24356964374999279, 195.6218750006145228, -15.72908226750539207 ) ) ;
#22753=CARTESIAN_POINT ( 'NONE',  ( -27.00000000000000355, 198.3125000012290400, 0.000000000000000000 ) ) ;
#22773=CYLINDRICAL_SURFACE ( 'NONE', #20352, 27.00000000000000355 ) ;
#22800=ADVANCED_FACE ( 'NONE', ( #22326 ), #27999, .T. ) ;
#22801=CARTESIAN_POINT ( 'NONE',  ( -20.86978606573367045, 194.8588513912095266, -17.51182790300216752 ) ) ;
#22803=CARTESIAN_POINT ( 'NONE',  ( -27.00000000000000355, 196.8125000000000000, -15.58845726811989429 ) ) ;
#22814=CARTESIAN_POINT ( 'NONE',  ( 13.62178482187501416, 195.0031250006145456, 23.59362340125806767 ) ) ;
#22815=CARTESIAN_POINT ( 'NONE',  ( 27.24356964375000345, 197.3843750006145399, -3.336375036156643733E-15 ) ) ;
#22817=CARTESIAN_POINT ( 'NONE',  ( -27.00000000000000355, 198.6500000000000341, 0.000000000000000000 ) ) ;
#22825=CARTESIAN_POINT ( 'NONE',  ( 1.120210788295102201E-13, 195.8375000000000057, -27.00000000000000711 ) ) ;
#22834=CARTESIAN_POINT ( 'NONE',  ( -27.00000000000000355, 195.0263594417697846, -9.827195513778322677 ) ) ;
#22836=VERTEX_POINT ( 'NONE', #16269 ) ;
#22840=ADVANCED_BREP_SHAPE_REPRESENTATION ( '', ( #7452, #17215 ), #33555 ) ;
#22848=( BOUNDED_CURVE ( )  B_SPLINE_CURVE ( 2, ( #12511, #15544, #29748, #3970, #24630, #24075, #18207, #24264, #9666 ),
 .UNSPECIFIED., .F., .F. ) 
 B_SPLINE_CURVE_WITH_KNOTS ( ( 3, 2, 2, 2, 3 ),
 ( 0.1041666666666666713, 0.1111111111111111049, 0.1250000000000000000, 0.1388888888888888951, 0.1458333333333333426 ),
 .UNSPECIFIED. ) 
 CURVE ( )  GEOMETRIC_REPRESENTATION_ITEM ( )  RATIONAL_B_SPLINE_CURVE ( ( 0.9330127018922194093, 0.9330127018922194093, 1.000000000000000000, 0.8660254037844387076, 1.000000000000000000, 0.8660254037844387076, 1.000000000000000000, 0.9330127018922194093, 0.9330127018922194093 ) ) 
 REPRESENTATION_ITEM ( '' )  );
#22871=CARTESIAN_POINT ( 'NONE',  ( -26.99999999999999645, 197.9000000012290457, 15.58845726811991561 ) ) ;
#22908=VECTOR ( 'NONE', #24718, 1000.000000000000227 ) ;
#22918=CARTESIAN_POINT ( 'NONE',  ( -27.00000000000000355, 197.2624999999999886, -15.58845726811989429 ) ) ;
#22940=CARTESIAN_POINT ( 'NONE',  ( -27.00000000000000355, 197.4125000012290343, 0.000000000000000000 ) ) ;
#22955=CARTESIAN_POINT ( 'NONE',  ( 27.00000000000001421, 196.7000000012290286, 15.58845726811988897 ) ) ;
#22968=CARTESIAN_POINT ( 'NONE',  ( -27.24356964374999279, 198.5468750006145342, 15.72908226750539384 ) ) ;
#22970=ORIENTED_EDGE ( 'NONE', *, *, #12890, .F. ) ;
#22978=CARTESIAN_POINT ( 'NONE',  ( 27.24356964374999635, 199.6156250006145285, -15.72908226750539029 ) ) ;
#22997=CARTESIAN_POINT ( 'NONE',  ( -27.24356964374999635, 195.8468750006145171, 15.72908226750539384 ) ) ;
#23015=CARTESIAN_POINT ( 'NONE',  ( -1.926257025242585782E-15, 199.7468750006145513, -31.45816453501075927 ) ) ;
#23020=ORIENTED_EDGE ( 'NONE', *, *, #25391, .T. ) ;
#23023=DIRECTION ( 'NONE',  ( -0.000000000000000000, -1.000000000000000000, -0.000000000000000000 ) ) ;
#23054=CARTESIAN_POINT ( 'NONE',  ( -7.234628195640289583, 197.7700961906613770, -27.00000000000001421 ) ) ;
#23064=CARTESIAN_POINT ( 'NONE',  ( -27.00000000000000355, 196.4750000012289775, -15.58845726811989429 ) ) ;
#23122=CARTESIAN_POINT ( 'NONE',  ( -13.49999999999998401, 195.6875000012290400, 23.38268590217985476 ) ) ;
#23139=CARTESIAN_POINT ( 'NONE',  ( 27.00000000000000355, 196.7375000012290229, -3.306546357697854128E-15 ) ) ;
#23148=EDGE_CURVE ( 'NONE', #25162, #36971, #28203, .T. ) ;
#23163=EDGE_LOOP ( 'NONE', ( #28234, #21352 ) ) ;
#23165=CARTESIAN_POINT ( 'NONE',  ( 27.24356964375000700, 198.1906250006145740, 15.72908226750537075 ) ) ;
#23183=CARTESIAN_POINT ( 'NONE',  ( -13.49999999999998401, 198.8375000012290457, 23.38268590217985476 ) ) ;
#23184=CARTESIAN_POINT ( 'NONE',  ( -27.24356964375000345, 195.8093750006145513, 0.000000000000000000 ) ) ;
#23193=ORIENTED_EDGE ( 'NONE', *, *, #23790, .T. ) ;
#23203=CARTESIAN_POINT ( 'NONE',  ( 5.727106289114498080E-15, 195.1625000000000227, 31.17691453623979214 ) ) ;
#23231=CARTESIAN_POINT ( 'NONE',  ( -27.24356964375000345, 199.7656250006145342, -15.72908226750537786 ) ) ;
#23281=CARTESIAN_POINT ( 'NONE',  ( -13.49999999999998401, 197.0375000012290627, 23.38268590217985476 ) ) ;
#23287=LINE ( 'NONE', #9251, #31098 ) ;
#23307=CARTESIAN_POINT ( 'NONE',  ( -1.909035429704832693E-15, 196.8500000012290343, -31.17691453623979214 ) ) ;
#23322=CARTESIAN_POINT ( 'NONE',  ( 5.778771075727756162E-15, 196.3718750006145513, 31.45816453501075927 ) ) ;
#23332=DIRECTION ( 'NONE',  ( 0.000000000000000000, -1.000000000000000000, 0.000000000000000000 ) ) ;
#23335=CARTESIAN_POINT ( 'NONE',  ( -13.62178482187500528, 199.7843750006145456, -23.59362340125807123 ) ) ;
#23360=EDGE_CURVE ( 'NONE', #36105, #5013, #6366, .T. ) ;
#23368=CARTESIAN_POINT ( 'NONE',  ( -27.24356964375000345, 196.7093750006145569, 0.000000000000000000 ) ) ;
#23385=CARTESIAN_POINT ( 'NONE',  ( -27.24356964374999990, 197.1218750006145228, -15.72908226750537786 ) ) ;
#23390=CARTESIAN_POINT ( 'NONE',  ( -13.50000000000000533, 195.4250000000000114, -23.38268590217984411 ) ) ;
#23442=VECTOR ( 'NONE', #28284, 1000.000000000000000 ) ;
#23474=CARTESIAN_POINT ( 'NONE',  ( 26.99999999999999645, 196.6625000000000512, -15.58845726811990495 ) ) ;
#23488=CARTESIAN_POINT ( 'NONE',  ( 27.00000000000000355, 196.7375000012290229, -3.306546357697854128E-15 ) ) ;
#23491=ADVANCED_FACE ( 'NONE', ( #9587 ), #18813, .F. ) ;
#23521=CARTESIAN_POINT ( 'NONE',  ( 26.99999999999999645, 198.9125000000000512, -15.58845726811990495 ) ) ;
#23523=CARTESIAN_POINT ( 'NONE',  ( 27.24356964375000700, 199.1468750006145285, 15.72908226750537075 ) ) ;
#23534=CARTESIAN_POINT ( 'NONE',  ( -1.926257025242585782E-15, 198.3406250006145228, -31.45816453501075927 ) ) ;
#23558=CARTESIAN_POINT ( 'NONE',  ( 13.62178482187501416, 195.5093750006145399, 23.59362340125806767 ) ) ;
#23559=CARTESIAN_POINT ( 'NONE',  ( 5.438367727407757144E-14, 198.2000000012290002, -27.00000000000000000 ) ) ;
#23560=CARTESIAN_POINT ( 'NONE',  ( -13.49999999999998401, 198.7250000000000227, 23.38268590217985476 ) ) ;
#23574=CARTESIAN_POINT ( 'NONE',  ( 13.62178482187499640, 198.8093750006145513, -23.59362340125807123 ) ) ;
#23619=CARTESIAN_POINT ( 'NONE',  ( 27.00000000000000355, 198.8750000000000284, -3.306546357697854128E-15 ) ) ;
#23635=DIRECTION ( 'NONE',  ( 0.000000000000000000, 0.000000000000000000, -1.000000000000000000 ) ) ;
#23678=CARTESIAN_POINT ( 'NONE',  ( 26.99999999999999645, 196.7750000012290741, -15.58845726811990495 ) ) ;
#23700=CARTESIAN_POINT ( 'NONE',  ( 5.778771075727756162E-15, 195.9218750006145342, 31.45816453501075927 ) ) ;
#23710=DIRECTION ( 'NONE',  ( 0.000000000000000000, 0.000000000000000000, -1.000000000000000000 ) ) ;
#23712=CARTESIAN_POINT ( 'NONE',  ( 27.24356964375000345, 199.1843750006145228, -3.336375036156643733E-15 ) ) ;
#23725=CARTESIAN_POINT ( 'NONE',  ( 13.62178482187501416, 198.6031250006145399, 23.59362340125806767 ) ) ;
#23747=CARTESIAN_POINT ( 'NONE',  ( -27.24356964375001056, 194.8857344423495874, -9.915847621322177119 ) ) ;
#23762=CARTESIAN_POINT ( 'NONE',  ( 27.24356964375000345, 197.3843750006145399, -3.336375036156643733E-15 ) ) ;
#23763=ORIENTED_EDGE ( 'NONE', *, *, #19158, .F. ) ;
#23790=EDGE_CURVE ( 'NONE', #25286, #16548, #11036, .T. ) ;
#23803=CARTESIAN_POINT ( 'NONE',  ( -3.253724281355068545E-15, 197.6374999999999602, -27.00000000000000000 ) ) ;
#23810=ORIENTED_EDGE ( 'NONE', *, *, #26862, .T. ) ;
#23812=CARTESIAN_POINT ( 'NONE',  ( -4.694659320240884604E-14, 197.4124999999999943, 27.00000000000000000 ) ) ;
#23827=SHAPE_DEFINITION_REPRESENTATION ( #17744, #10836 ) ;
#23871=CARTESIAN_POINT ( 'NONE',  ( -20.68320086892770604, 194.6619763917542514, -17.35526438333879540 ) ) ;
#23888=CARTESIAN_POINT ( 'NONE',  ( -13.49999999999998401, 199.1750000000000114, 23.38268590217985476 ) ) ;
#23892=CARTESIAN_POINT ( 'NONE',  ( -27.24356964374999635, 195.3968750006145569, 15.72908226750539384 ) ) ;
#23897=CARTESIAN_POINT ( 'NONE',  ( 0.000000000000000000, 0.000000000000000000, -5.000000000000000000 ) ) ;
#23901=CARTESIAN_POINT ( 'NONE',  ( 26.99999999999999645, 198.4625000000000057, -15.58845726811990495 ) ) ;
#23903=CARTESIAN_POINT ( 'NONE',  ( -27.24356964375000345, 197.1593750006145456, 0.000000000000000000 ) ) ;
#23911=( BOUNDED_CURVE ( )  B_SPLINE_CURVE ( 2, ( #15566, #12717, #9688, #21079, #958 ),
 .UNSPECIFIED., .F., .F. ) 
 B_SPLINE_CURVE_WITH_KNOTS ( ( 3, 2, 3 ),
 ( 0.000000000000000000, 0.01388888888888888985, 0.02083333333333333565 ),
 .UNSPECIFIED. ) 
 CURVE ( )  GEOMETRIC_REPRESENTATION_ITEM ( )  RATIONAL_B_SPLINE_CURVE ( ( 1.000000000000000000, 0.8660254037844387076, 1.000000000000000000, 0.9330127018922192983, 0.9330127018922194093 ) ) 
 REPRESENTATION_ITEM ( '' )  );
#23916=CARTESIAN_POINT ( 'NONE',  ( -27.24356964374999635, 195.7906250006145115, 15.72908226750539384 ) ) ;
#23938=CARTESIAN_POINT ( 'NONE',  ( -27.24356964375000345, 198.9031250006145228, 0.000000000000000000 ) ) ;
#23953=CARTESIAN_POINT ( 'NONE',  ( -27.24356964374999990, 198.9218750006145626, -15.72908226750537786 ) ) ;
#23981=CARTESIAN_POINT ( 'NONE',  ( -13.62178482187498396, 196.7281250006145399, 23.59362340125808188 ) ) ;
#23982=EDGE_CURVE ( 'NONE', #28452, #36517, #29137, .T. ) ;
#23997=CARTESIAN_POINT ( 'NONE',  ( 27.00000000000001066, 199.2875000000000227, 15.58845726811988897 ) ) ;
#24000=VERTEX_POINT ( 'NONE', #17606 ) ;
#24015=EDGE_CURVE ( 'NONE', #4383, #15329, #34288, .T. ) ;
#24023=ORIENTED_EDGE ( 'NONE', *, *, #14020, .F. ) ;
#24036=LINE ( 'NONE', #7167, #20223 ) ;
#24056=CARTESIAN_POINT ( 'NONE',  ( 27.00000000000001066, 195.3500000012290343, 15.58845726811988897 ) ) ;
#24075=CARTESIAN_POINT ( 'NONE',  ( 27.00000000000001421, 198.9500000012290002, 15.58845726811988897 ) ) ;
#24077=CARTESIAN_POINT ( 'NONE',  ( -27.24356964374999990, 196.2218750006145456, -15.72908226750537786 ) ) ;
#24086=CARTESIAN_POINT ( 'NONE',  ( 13.49999999999999645, 198.9500000000000171, -23.38268590217984766 ) ) ;
#24088=CARTESIAN_POINT ( 'NONE',  ( 13.62178482187501416, 196.4093750006145456, 23.59362340125806767 ) ) ;
#24102=CARTESIAN_POINT ( 'NONE',  ( 27.24356964374999635, 196.4656250006145228, -15.72908226750539029 ) ) ;
#24127=CARTESIAN_POINT ( 'NONE',  ( -27.24356964375000345, 199.3531250006145399, 0.000000000000000000 ) ) ;
#24157=CARTESIAN_POINT ( 'NONE',  ( 5.438367727407757144E-14, 198.0875000000000057, -27.00000000000000000 ) ) ;
#24164=CARTESIAN_POINT ( 'NONE',  ( -1.926257025242585782E-15, 197.8906250006145342, -31.45816453501076637 ) ) ;
#24181=CARTESIAN_POINT ( 'NONE',  ( -27.00000000000000355, 199.9625000000000341, -15.58845726811989429 ) ) ;
#24196=CARTESIAN_POINT ( 'NONE',  ( -27.24356964375000345, 199.8312500006145171, 0.000000000000000000 ) ) ;
#24216=CARTESIAN_POINT ( 'NONE',  ( 1.069080835302379631E-14, 198.8750000012290400, 27.00000000000000000 ) ) ;
#24264=CARTESIAN_POINT ( 'NONE',  ( 7.234628195640322446, 198.8950961906613770, 26.99999999999999645 ) ) ;
#24278=CARTESIAN_POINT ( 'NONE',  ( 5.778771075727756162E-15, 197.2718750006145569, 31.45816453501076637 ) ) ;
#24291=CARTESIAN_POINT ( 'NONE',  ( -27.24356964374999635, 195.3406250006145513, 15.72908226750539384 ) ) ;
#24315=CARTESIAN_POINT ( 'NONE',  ( 13.62178482187501416, 199.0531250006145285, 23.59362340125806767 ) ) ;
#24347=CARTESIAN_POINT ( 'NONE',  ( -26.99999999999999645, 198.2375000000000114, 15.58845726811991561 ) ) ;
#24355=CARTESIAN_POINT ( 'NONE',  ( 27.24356964375000700, 198.6406250006145342, 15.72908226750537075 ) ) ;
#24357=CARTESIAN_POINT ( 'NONE',  ( -1.045839947578415010E-13, 194.8250000012290570, 27.00000000000000355 ) ) ;
#24369=CARTESIAN_POINT ( 'NONE',  ( 27.00000000000000355, 197.9750000000000227, -3.306546357697854128E-15 ) ) ;
#24377=CARTESIAN_POINT ( 'NONE',  ( -3.253724281355068545E-15, 196.2874999999999659, -27.00000000000000000 ) ) ;
#24395=CARTESIAN_POINT ( 'NONE',  ( -27.00000000000000355, 196.0250000012290457, -15.58845726811989429 ) ) ;
#24462=CARTESIAN_POINT ( 'NONE',  ( 5.778771075727756162E-15, 198.1718750006145342, 31.45816453501076637 ) ) ;
#24476=CARTESIAN_POINT ( 'NONE',  ( 27.24356964375000345, 196.4281250006145569, -3.336375036156643733E-15 ) ) ;
#24486=ORIENTED_EDGE ( 'NONE', *, *, #29019, .F. ) ;
#24487=CARTESIAN_POINT ( 'NONE',  ( -27.00000000000000355, 195.1250000012290400, -15.58845726811989429 ) ) ;
#24501=CARTESIAN_POINT ( 'NONE',  ( 27.24356964375000700, 199.5406250006145683, 15.72908226750537075 ) ) ;
#24503=LINE ( 'NONE', #32645, #10167 ) ;
#24521=ADVANCED_FACE ( 'NONE', ( #35250, #17844 ), #6266, .F. ) ;
#24525=CARTESIAN_POINT ( 'NONE',  ( 0.000000000000000000, 2.000000000000000000, -25.00000000000000000 ) ) ;
#24536=CARTESIAN_POINT ( 'NONE',  ( 13.62178482187501416, 196.8031250006145285, 23.59362340125806767 ) ) ;
#24552=CARTESIAN_POINT ( 'NONE',  ( -1.909035429704832693E-15, 197.6375000000000171, -31.17691453623979214 ) ) ;
#24623=CARTESIAN_POINT ( 'NONE',  ( 1.120210788295102201E-13, 195.0500000012290513, -27.00000000000000711 ) ) ;
#24630=CARTESIAN_POINT ( 'NONE',  ( 27.00000000000000355, 198.9875000012290229, -3.306546357697854128E-15 ) ) ;
#24642=CARTESIAN_POINT ( 'NONE',  ( -1.926257025242585782E-15, 197.4968750006145513, -31.45816453501076637 ) ) ;
#24650=VERTEX_POINT ( 'NONE', #26722 ) ;
#24653=CARTESIAN_POINT ( 'NONE',  ( 27.24356964375000700, 196.8406250006145513, 15.72908226750537075 ) ) ;
#24666=DIRECTION ( 'NONE',  ( 0.000000000000000000, 0.000000000000000000, -1.000000000000000000 ) ) ;
#24678=CARTESIAN_POINT ( 'NONE',  ( 13.62178482187499640, 196.9531250006145342, -23.59362340125807123 ) ) ;
#24705=CARTESIAN_POINT ( 'NONE',  ( 1.069080835302379631E-14, 196.9624999999999773, 27.00000000000000000 ) ) ;
#24714=ORIENTED_EDGE ( 'NONE', *, *, #36536, .F. ) ;
#24717=CARTESIAN_POINT ( 'NONE',  ( 27.24356964374999279, 196.4656250006145797, -15.72908226750539207 ) ) ;
#24718=DIRECTION ( 'NONE',  ( -0.8660254037844613562, -0.4999999999999605871, 0.000000000000000000 ) ) ;
#24727=CARTESIAN_POINT ( 'NONE',  ( -1.045839947578415010E-13, 196.5125000000000455, 27.00000000000000355 ) ) ;
#24733=CARTESIAN_POINT ( 'NONE',  ( 27.00000000000001066, 197.9375000000000284, 15.58845726811988897 ) ) ;
#24762=DIRECTION ( 'NONE',  ( 0.000000000000000000, 0.000000000000000000, -1.000000000000000000 ) ) ;
#24826=CARTESIAN_POINT ( 'NONE',  ( 27.24356964375000345, 195.1343750006145399, -3.336375036156643733E-15 ) ) ;
#24839=CARTESIAN_POINT ( 'NONE',  ( 5.727106289114498080E-15, 197.9750000012290343, 31.17691453623979214 ) ) ;
#24840=VECTOR ( 'NONE', #29681, 1000.000000000000000 ) ;
#24866=CARTESIAN_POINT ( 'NONE',  ( 13.62178482187499640, 196.0531250006145285, -23.59362340125807123 ) ) ;
#24900=CARTESIAN_POINT ( 'NONE',  ( -27.00000000000000355, 197.4125000012290343, 0.000000000000000000 ) ) ;
#24904=CARTESIAN_POINT ( 'NONE',  ( 27.24356964374999635, 198.3218750006145399, -15.72908226750539029 ) ) ;
#24918=CARTESIAN_POINT ( 'NONE',  ( 27.00000000000001066, 197.0374999999999943, 15.58845726811988897 ) ) ;
#24999=CYLINDRICAL_SURFACE ( 'NONE', #16200, 27.00000000000000355 ) ;
#25011=CARTESIAN_POINT ( 'NONE',  ( 27.24356964374999279, 195.1718750006145342, -15.72908226750539207 ) ) ;
#25023=CARTESIAN_POINT ( 'NONE',  ( 13.62178482187499640, 195.1531250006145513, -23.59362340125807123 ) ) ;
#25039=CARTESIAN_POINT ( 'NONE',  ( 27.00000000000001421, 199.2874999999999943, 15.58845726811988897 ) ) ;
#25044=MECHANICAL_DESIGN_GEOMETRIC_PRESENTATION_REPRESENTATION('',(#34135),#3257);
#25049=CARTESIAN_POINT ( 'NONE',  ( 13.62178482187501416, 195.9031250006145513, 23.59362340125806767 ) ) ;
#25069=AXIS2_PLACEMENT_3D ( 'NONE', #2577, #34418, #25700 ) ;
#25088=CARTESIAN_POINT ( 'NONE',  ( -27.24356964375000345, 196.1656250006145399, -15.72908226750537786 ) ) ;
#25089=CARTESIAN_POINT ( 'NONE',  ( -27.24356964374999990, 198.0218750006145569, -15.72908226750537786 ) ) ;
#25104=CARTESIAN_POINT ( 'NONE',  ( 27.00000000000000355, 196.6250000000000284, -3.306546357697854128E-15 ) ) ;
#25112=CARTESIAN_POINT ( 'NONE',  ( -7.234628195640307347, 199.1200961906613713, -27.00000000000000711 ) ) ;
#25162=VERTEX_POINT ( 'NONE', #21167 ) ;
#25192=CARTESIAN_POINT ( 'NONE',  ( -7.234628195640263826, 197.2075961894323370, -27.00000000000003553 ) ) ;
#25204=CARTESIAN_POINT ( 'NONE',  ( -27.24356964375000345, 195.8093750006145513, 0.000000000000000000 ) ) ;
#25216=CARTESIAN_POINT ( 'NONE',  ( -26.99999999999998934, 199.2500000012290116, 15.58845726811991561 ) ) ;
#25237=CARTESIAN_POINT ( 'NONE',  ( 5.778771075727756162E-15, 194.9656250006145228, 31.45816453501075927 ) ) ;
#25278=CARTESIAN_POINT ( 'NONE',  ( -13.62178482187498396, 199.0343750006145456, 23.59362340125808188 ) ) ;
#25281=FACE_OUTER_BOUND ( 'NONE', #1150, .T. ) ;
#25286=VERTEX_POINT ( 'NONE', #23812 ) ;
#25293=CARTESIAN_POINT ( 'NONE',  ( -27.24356964374999635, 198.9968750006145228, 15.72908226750539384 ) ) ;
#25317=( BOUNDED_CURVE ( )  B_SPLINE_CURVE ( 2, ( #19890, #34459, #23281, #8500, #20068, #17410, #25929, #31613, #37473 ),
 .UNSPECIFIED., .F., .F. ) 
 B_SPLINE_CURVE_WITH_KNOTS ( ( 3, 2, 2, 2, 3 ),
 ( 0.4791666666666666852, 0.4861111111111111049, 0.5000000000000000000, 0.5138888888888888395, 0.5208333333333333703 ),
 .UNSPECIFIED. ) 
 CURVE ( )  GEOMETRIC_REPRESENTATION_ITEM ( )  RATIONAL_B_SPLINE_CURVE ( ( 0.9330127018922194093, 0.9330127018922196314, 1.000000000000000000, 0.8660254037844387076, 1.000000000000000000, 0.8660254037844387076, 1.000000000000000000, 0.9330127018922187432, 0.9330127018922192983 ) ) 
 REPRESENTATION_ITEM ( '' )  );
#25383=LINE ( 'NONE', #10603, #20482 ) ;
#25391=EDGE_CURVE ( 'NONE', #9546, #24650, #2974, .T. ) ;
#25398=CARTESIAN_POINT ( 'NONE',  ( -27.00000000000000355, 197.8250000012290286, -15.58845726811989429 ) ) ;
#25423=CARTESIAN_POINT ( 'NONE',  ( -27.24356964374999635, 197.1406250006145058, 15.72908226750539384 ) ) ;
#25448=FACE_OUTER_BOUND ( 'NONE', #813, .T. ) ;
#25462=CARTESIAN_POINT ( 'NONE',  ( -20.86978604919638869, 194.8026013911397456, -17.51182792271053046 ) ) ;
#25463=CARTESIAN_POINT ( 'NONE',  ( -13.62178482187500528, 198.8843750006145399, -23.59362340125807123 ) ) ;
#25466=CARTESIAN_POINT ( 'NONE',  ( 13.50000000000001421, 195.6500000000000057, 23.38268590217984055 ) ) ;
#25478=CARTESIAN_POINT ( 'NONE',  ( -27.24356964374999635, 199.4468750006145399, 15.72908226750539384 ) ) ;
#25481=ORIENTED_EDGE ( 'NONE', *, *, #5298, .T. ) ;
#25491=( NAMED_UNIT ( * ) SI_UNIT ( $, .STERADIAN. ) SOLID_ANGLE_UNIT ( ) );
#25539=CARTESIAN_POINT ( 'NONE',  ( -26.99999999999999645, 199.5875000000000341, 15.58845726811991561 ) ) ;
#25582=CARTESIAN_POINT ( 'NONE',  ( 5.727106289114498080E-15, 198.8750000012290400, 31.17691453623979214 ) ) ;
#25606=DIRECTION ( 'NONE',  ( 0.000000000000000000, 1.000000000000000000, 0.000000000000000000 ) ) ;
#25613=EDGE_LOOP ( 'NONE', ( #16057, #3476, #1547, #12734 ) ) ;
#25645=CARTESIAN_POINT ( 'NONE',  ( 13.62178482187501416, 198.2093750006145285, 23.59362340125806767 ) ) ;
#25655=CARTESIAN_POINT ( 'NONE',  ( -27.00000000000000355, 195.9125000000000796, -15.58845726811989429 ) ) ;
#25662=CARTESIAN_POINT ( 'NONE',  ( -27.00000000000000355, 195.4625000000000057, -15.58845726811989429 ) ) ;
#25675=AXIS2_PLACEMENT_3D ( 'NONE', #12338, #9503, #15188 ) ;
#25700=DIRECTION ( 'NONE',  ( 1.000000000000000000, 0.000000000000000000, 0.000000000000000000 ) ) ;
#25766=CARTESIAN_POINT ( 'NONE',  ( -27.00000000000000355, 196.9250000012290229, -15.58845726811989429 ) ) ;
#25778=CYLINDRICAL_SURFACE ( 'NONE', #226, 5.000000000000000000 ) ;
#25782=CARTESIAN_POINT ( 'NONE',  ( 7.234628195640363302, 196.8299038117967257, -26.99999999999996803 ) ) ;
#25786=ORIENTED_EDGE ( 'NONE', *, *, #29045, .T. ) ;
#25796=CARTESIAN_POINT ( 'NONE',  ( -13.62178482187498396, 198.5843750006145569, 23.59362340125808188 ) ) ;
#25808=CARTESIAN_POINT ( 'NONE',  ( -27.00000000000000355, 200.0000000000000000, 0.000000000000000000 ) ) ;
#25810=ADVANCED_FACE ( 'NONE', ( #5568 ), #11454, .T. ) ;
#25820=CARTESIAN_POINT ( 'NONE',  ( -27.00000000000000355, 196.8500000000000227, 0.000000000000000000 ) ) ;
#25830=CARTESIAN_POINT ( 'NONE',  ( -27.24356964374999635, 196.7468750006145797, 15.72908226750539384 ) ) ;
#25838=ORIENTED_EDGE ( 'NONE', *, *, #23360, .T. ) ;
#25843=VERTEX_POINT ( 'NONE', #17336 ) ;
#25850=CARTESIAN_POINT ( 'NONE',  ( 27.24356964375000345, 199.1843750006145228, -3.336375036156643733E-15 ) ) ;
#25898=CARTESIAN_POINT ( 'NONE',  ( -7.234628195640302017, 196.6049038117967029, 27.00000000000000711 ) ) ;
#25915=CARTESIAN_POINT ( 'NONE',  ( 0.000000000000000000, 200.0000000000000000, -27.00000000000000355 ) ) ;
#25929=CARTESIAN_POINT ( 'NONE',  ( -13.50000000000000533, 196.8875000012290286, -23.38268590217984411 ) ) ;
#25935=CARTESIAN_POINT ( 'NONE',  ( -3.253724281355068545E-15, 198.6500000012290172, -27.00000000000000000 ) ) ;
#25955=CARTESIAN_POINT ( 'NONE',  ( -26.99999999999998934, 196.1000000012290627, 15.58845726811991561 ) ) ;
#25975=CARTESIAN_POINT ( 'NONE',  ( -27.24356964375001056, 194.8294844423495533, -9.915847621322177119 ) ) ;
#25983=CARTESIAN_POINT ( 'NONE',  ( 27.24356964375000700, 199.5968750006145740, 15.72908226750537075 ) ) ;
#25993=CARTESIAN_POINT ( 'NONE',  ( 27.24356964375000700, 199.0906250006145228, 15.72908226750537075 ) ) ;
#25994=EDGE_CURVE ( 'NONE', #36517, #36421, #4416, .T. ) ;
#26004=EDGE_LOOP ( 'NONE', ( #9350, #37030, #7411, #32096 ) ) ;
#26005=PLANE ( 'NONE',  #22192 ) ;
#26016=CARTESIAN_POINT ( 'NONE',  ( 27.24356964374999635, 196.0718750006145683, -15.72908226750539029 ) ) ;
#26033=CARTESIAN_POINT ( 'NONE',  ( 27.24356964374999635, 199.6718750006145058, -15.72908226750539029 ) ) ;
#26034=VERTEX_POINT ( 'NONE', #5499 ) ;
#26064=CARTESIAN_POINT ( 'NONE',  ( 27.24356964375000345, 199.1281250006145171, -3.336375036156643733E-15 ) ) ;
#26106=CARTESIAN_POINT ( 'NONE',  ( 1.069080835302379631E-14, 199.2125000000000057, 27.00000000000000000 ) ) ;
#26115=DIRECTION ( 'NONE',  ( -0.000000000000000000, -1.000000000000000000, -0.000000000000000000 ) ) ;
#26116=CARTESIAN_POINT ( 'NONE',  ( 13.49999999999999645, 198.6125000012290513, -23.38268590217984766 ) ) ;
#26117=ORIENTED_EDGE ( 'NONE', *, *, #12493, .F. ) ;
#26129=ORIENTED_EDGE ( 'NONE', *, *, #13142, .F. ) ;
#26136=CARTESIAN_POINT ( 'NONE',  ( 13.49999999999999645, 197.7125000012290172, -23.38268590217984766 ) ) ;
#26158=DIRECTION ( 'NONE',  ( -0.000000000000000000, -1.000000000000000000, -0.000000000000000000 ) ) ;
#26167=CARTESIAN_POINT ( 'NONE',  ( -27.24356964375000345, 199.8218750006145399, -15.72908226750537786 ) ) ;
#26177=CARTESIAN_POINT ( 'NONE',  ( 27.24356964374999635, 198.2656250006145058, -15.72908226750539029 ) ) ;
#26196=CARTESIAN_POINT ( 'NONE',  ( 27.00000000000000355, 195.2750000000000057, -3.306546357697854128E-15 ) ) ;
#26197=CARTESIAN_POINT ( 'NONE',  ( 13.62178482187499640, 195.2093750006145569, -23.59362340125807123 ) ) ;
#26206=ORIENTED_EDGE ( 'NONE', *, *, #29259, .F. ) ;
#26214=CARTESIAN_POINT ( 'NONE',  ( 5.778771075727756162E-15, 198.6218750006145513, 31.45816453501075927 ) ) ;
#26220=CARTESIAN_POINT ( 'NONE',  ( -26.99999999999999645, 195.5374999999999943, 15.58845726811991561 ) ) ;
#26311=ORIENTED_EDGE ( 'NONE', *, *, #32089, .F. ) ;
#26320=CARTESIAN_POINT ( 'NONE',  ( 26.99999999999999645, 195.8750000012290400, -15.58845726811990495 ) ) ;
#26352=CARTESIAN_POINT ( 'NONE',  ( 13.62178482187501416, 199.5593750006145513, 23.59362340125806767 ) ) ;
#26363=CARTESIAN_POINT ( 'NONE',  ( 5.778771075727756162E-15, 198.5656250006145171, 31.45816453501075927 ) ) ;
#26381=EDGE_LOOP ( 'NONE', ( #26206, #23020, #21540, #27185 ) ) ;
#26386=CARTESIAN_POINT ( 'NONE',  ( -13.62178482187500528, 197.0843750006145285, -23.59362340125807123 ) ) ;
#26387=CARTESIAN_POINT ( 'NONE',  ( 13.50000000000001421, 198.0125000012290286, 23.38268590217984055 ) ) ;
#26389=EDGE_CURVE ( 'NONE', #32692, #22009, #35563, .T. ) ;
#26405=CARTESIAN_POINT ( 'NONE',  ( 27.24356964375000700, 197.3468750006145740, 15.72908226750537075 ) ) ;
#26499=ORIENTED_EDGE ( 'NONE', *, *, #12862, .F. ) ;
#26508=CARTESIAN_POINT ( 'NONE',  ( -26.99999999999998934, 197.4500000012290570, 15.58845726811991561 ) ) ;
#26519=DIRECTION ( 'NONE',  ( 0.000000000000000000, 0.000000000000000000, -1.000000000000000000 ) ) ;
#26528=CARTESIAN_POINT ( 'NONE',  ( -13.62178482187500528, 196.1843750006145228, -23.59362340125807123 ) ) ;
#26540=CARTESIAN_POINT ( 'NONE',  ( 27.24356964374999279, 199.6718750006145058, -15.72908226750539207 ) ) ;
#26552=CARTESIAN_POINT ( 'NONE',  ( 13.62178482187499640, 197.8531250006145399, -23.59362340125807123 ) ) ;
#26575=CARTESIAN_POINT ( 'NONE',  ( -27.24356964374999635, 194.9468750006145399, 15.72908226750539384 ) ) ;
#26577=CARTESIAN_POINT ( 'NONE',  ( -7.234628195640302017, 198.7424038105676800, 27.00000000000000711 ) ) ;
#26578=CARTESIAN_POINT ( 'NONE',  ( -27.00000000000000711, 195.0263594398178100, -9.827196325189913040 ) ) ;
#26583=VERTEX_POINT ( 'NONE', #24525 ) ;
#26591=CARTESIAN_POINT ( 'NONE',  ( 27.24356964374999635, 198.3218750006145399, -15.72908226750539029 ) ) ;
#26598=EDGE_CURVE ( 'NONE', #2631, #15329, #7463, .T. ) ;
#26670=CYLINDRICAL_SURFACE ( 'NONE', #26739, 25.00000000000000000 ) ;
#26673=CARTESIAN_POINT ( 'NONE',  ( 27.00000000000000355, 199.7750000000000057, -3.306546357697854128E-15 ) ) ;
#26716=CARTESIAN_POINT ( 'NONE',  ( -13.62178482187498396, 195.8843750006145399, 23.59362340125808188 ) ) ;
#26722=CARTESIAN_POINT ( 'NONE',  ( 1.255007937094097924E-14, 199.1000000012290627, -27.00000000000000355 ) ) ;
#26723=CARTESIAN_POINT ( 'NONE',  ( 1.069080835302379631E-14, 199.3250000012290286, 27.00000000000000000 ) ) ;
#26725=CARTESIAN_POINT ( 'NONE',  ( 13.50000000000001421, 198.8000000000000114, 23.38268590217984055 ) ) ;
#26727=CARTESIAN_POINT ( 'NONE',  ( 13.62178482187499640, 197.0093750006145399, -23.59362340125807123 ) ) ;
#26739=AXIS2_PLACEMENT_3D ( 'NONE', #7161, #32361, #4118 ) ;
#26740=CARTESIAN_POINT ( 'NONE',  ( 5.778771075727756162E-15, 199.4656250006145797, 31.45816453501075927 ) ) ;
#26749=( BOUNDED_CURVE ( )  B_SPLINE_CURVE ( 2, ( #6538, #23231, #14883, #9007, #20395, #18111, #6350, #17920, #17730, #6156, #29465, #17362, #3500, #31247, #5276, #15069, #28903, #12219, #26064, #93, #11655, #20577, #29272, #34779, #29083, #3125, #3311, #14693, #33251, #16201, #840, #24355, #12785, #12408, #27187, #30031, #21144, #18491, #7291, #1403, #18865, #1027, #30223, #21702, #7475, #4622, #35708, #10312, #4064, #1212, #15636, #24164, #32682, #36267, #18681, #35897, #6920, #6726, #27000, #29839, #18299, #9940, #9759, #10129, #33434, #32873, #21520, #3875, #21334, #21884, #33066, #7111, #4249, #15449, #12979, #19054, #15823, #30412, #30605, #27373, #24536, #36085, #23981, #4435, #16016, #35526, #27564, #1593, #13161, #24717, #9570, #12600, #22444, #34179, #13911, #33991, #14092, #25088, #16754, #36829, #8035, #19243, #27750, #28302, #5362, #7850, #33813, #10494, #16387, #30784, #22073, #2148, #13533, #22261, #19974, #10682, #37198, #4989, #1780, #31517, #19423, #30973, #8224, #33625, #19609, #7665, #11057, #10871, #22814, #16572, #13729, #5178, #5542, #2340, #25462 ),
 .UNSPECIFIED., .F., .F. ) 
 B_SPLINE_CURVE_WITH_KNOTS ( ( 3, 2, 2, 2, 2, 2, 2, 2, 2, 2, 2, 2, 2, 2, 2, 2, 2, 2, 2, 2, 2, 2, 2, 2, 2, 2, 2, 2, 2, 2, 2, 2, 2, 2, 2, 2, 2, 2, 2, 2, 2, 2, 2, 2, 2, 2, 2, 2, 2, 2, 2, 2, 2, 2, 2, 2, 2, 2, 2, 2, 2, 2, 2, 2, 2, 2, 2, 3 ),
 ( 0.000000000000000000, 0.01388888888888888812, 0.02777777777777777624, 0.04166666666666666435, 0.05555555555555555247, 0.06944444444444444753, 0.08333333333333332871, 0.09722222222222222376, 0.1111111111111111049, 0.1250000000000000000, 0.1388888888888888951, 0.1527777777777777901, 0.1666666666666666574, 0.1805555555555555525, 0.1944444444444444475, 0.2083333333333333426, 0.2222222222222222099, 0.2361111111111111049, 0.2500000000000000000, 0.2638888888888888951, 0.2777777777777777901, 0.2916666666666666852, 0.3055555555555555802, 0.3194444444444444198, 0.3333333333333333148, 0.3472222222222222099, 0.3611111111111111049, 0.3750000000000000000, 0.3888888888888888951, 0.4027777777777777901, 0.4166666666666666852, 0.4305555555555555802, 0.4444444444444444198, 0.4583333333333333148, 0.4722222222222222099, 0.4861111111111111049, 0.5000000000000000000, 0.5138888888888888395, 0.5277777777777777901, 0.5416666666666666297, 0.5555555555555555802, 0.5694444444444444198, 0.5833333333333333703, 0.5972222222222222099, 0.6111111111111111605, 0.6250000000000000000, 0.6388888888888888395, 0.6527777777777777901, 0.6666666666666666297, 0.6805555555555555802, 0.6944444444444444198, 0.7083333333333333703, 0.7222222222222222099, 0.7361111111111111605, 0.7500000000000000000, 0.7638888888888888395, 0.7777777777777777901, 0.7916666666666666297, 0.8055555555555555802, 0.8194444444444444198, 0.8333333333333333703, 0.8472222222222222099, 0.8611111111111111605, 0.8750000000000000000, 0.8888888888888888395, 0.9027777777777777901, 0.9166666666666666297, 0.9258785558287928596 ),
 .UNSPECIFIED. ) 
 CURVE ( )  GEOMETRIC_REPRESENTATION_ITEM ( )  RATIONAL_B_SPLINE_CURVE ( ( 1.000000000000000000, 0.8660254037844387076, 1.000000000000000000, 0.8660254037844387076, 1.000000000000000000, 0.8660254037844387076, 1.000000000000000000, 0.8660254037844387076, 1.000000000000000000, 0.8660254037844387076, 1.000000000000000000, 0.8660254037844387076, 1.000000000000000000, 0.8660254037844387076, 1.000000000000000000, 0.8660254037844387076, 1.000000000000000000, 0.8660254037844387076, 1.000000000000000000, 0.8660254037844387076, 1.000000000000000000, 0.8660254037844387076, 1.000000000000000000, 0.8660254037844387076, 1.000000000000000000, 0.8660254037844387076, 1.000000000000000000, 0.8660254037844387076, 1.000000000000000000, 0.8660254037844387076, 1.000000000000000000, 0.8660254037844387076, 1.000000000000000000, 0.8660254037844387076, 1.000000000000000000, 0.8660254037844387076, 1.000000000000000000, 0.8660254037844387076, 1.000000000000000000, 0.8660254037844387076, 1.000000000000000000, 0.8660254037844387076, 1.000000000000000000, 0.8660254037844387076, 1.000000000000000000, 0.8660254037844387076, 1.000000000000000000, 0.8660254037844387076, 1.000000000000000000, 0.8660254037844387076, 1.000000000000000000, 0.8660254037844387076, 1.000000000000000000, 0.8660254037844387076, 1.000000000000000000, 0.8660254037844387076, 1.000000000000000000, 0.8660254037844387076, 1.000000000000000000, 0.8660254037844387076, 1.000000000000000000, 0.8660254037844387076, 1.000000000000000000, 0.8660254037844387076, 1.000000000000000000, 0.8660254037844387076, 1.000000000000000000, 0.8660254037844387076, 1.000000000000000000, 0.8660254037844387076, 1.000000000000000000, 0.8660254037844387076, 1.000000000000000000, 0.8660254037844387076, 1.000000000000000000, 0.8660254037844387076, 1.000000000000000000, 0.8660254037844387076, 1.000000000000000000, 0.8660254037844387076, 1.000000000000000000, 0.8660254037844387076, 1.000000000000000000, 0.8660254037844387076, 1.000000000000000000, 0.8660254037844387076, 1.000000000000000000, 0.8660254037844387076, 1.000000000000000000, 0.8660254037844387076, 1.000000000000000000, 0.8660254037844387076, 1.000000000000000000, 0.8660254037844387076, 1.000000000000000000, 0.8660254037844387076, 1.000000000000000000, 0.8660254037844387076, 1.000000000000000000, 0.8660254037844387076, 1.000000000000000000, 0.8660254037844387076, 1.000000000000000000, 0.8660254037844387076, 1.000000000000000000, 0.8660254037844387076, 1.000000000000000000, 0.8660254037844387076, 1.000000000000000000, 0.8660254037844387076, 1.000000000000000000, 0.8660254037844387076, 1.000000000000000000, 0.8660254037844387076, 1.000000000000000000, 0.8660254037844387076, 1.000000000000000000, 0.8660254037844387076, 1.000000000000000000, 0.8660254037844387076, 1.000000000000000000, 0.8660254037844387076, 1.000000000000000000, 0.8660254037844387076, 1.000000000000000000, 0.8660254037844387076, 1.000000000000000000, 0.8660254037844387076, 1.000000000000000000, 0.8660254037844387076, 1.000000000000000000, 0.8660254037844387076, 1.000000000000000000, 0.9111405425767590271, 0.9401542252352144136 ) ) 
 REPRESENTATION_ITEM ( '' )  );
#26752=VERTEX_POINT ( 'NONE', #19229 ) ;
#26766=CARTESIAN_POINT ( 'NONE',  ( -1.926257025242585782E-15, 198.7906250006145399, -31.45816453501075927 ) ) ;
#26782=CARTESIAN_POINT ( 'NONE',  ( 13.62178482187499640, 197.4593750006145285, -23.59362340125807123 ) ) ;
#26807=EDGE_CURVE ( 'NONE', #36105, #28452, #27673, .T. ) ;
#26826=FACE_OUTER_BOUND ( 'NONE', #14616, .T. ) ;
#26827=CARTESIAN_POINT ( 'NONE',  ( 13.49999999999999645, 199.8499999999999943, -23.38268590217984766 ) ) ;
#26862=EDGE_CURVE ( 'NONE', #25843, #37126, #14604, .T. ) ;
#26877=ADVANCED_FACE ( 'NONE', ( #34537 ), #26005, .T. ) ;
#26911=CARTESIAN_POINT ( 'NONE',  ( -27.24356964374999990, 195.7718750006145569, -15.72908226750537786 ) ) ;
#26913=ORIENTED_EDGE ( 'NONE', *, *, #31608, .F. ) ;
#26918=CARTESIAN_POINT ( 'NONE',  ( 1.069080835302379631E-14, 199.6625000000000227, 27.00000000000000000 ) ) ;
#26920=CARTESIAN_POINT ( 'NONE',  ( -27.24356964375000345, 196.6718750006145342, -15.72908226750537786 ) ) ;
#26932=CARTESIAN_POINT ( 'NONE',  ( -27.24356964374999635, 196.2406250006145285, 15.72908226750539384 ) ) ;
#26940=ADVANCED_FACE ( 'NONE', ( #25448 ), #34353, .T. ) ;
#26955=CARTESIAN_POINT ( 'NONE',  ( -13.62178482187500528, 199.2781250006145228, -23.59362340125807123 ) ) ;
#26974=APPLICATION_CONTEXT ( 'automotive_design' ) ;
#27000=CARTESIAN_POINT ( 'NONE',  ( -13.62178482187498396, 197.6281250006145171, 23.59362340125808188 ) ) ;
#27012=DIRECTION ( 'NONE',  ( -0.000000000000000000, -1.000000000000000000, -0.000000000000000000 ) ) ;
#27019=CARTESIAN_POINT ( 'NONE',  ( -13.50000000000000533, 199.0250000000000057, -23.38268590217984411 ) ) ;
#27044=CIRCLE ( 'NONE', #6479, 27.00000000000000355 ) ;
#27083=CARTESIAN_POINT ( 'NONE',  ( -26.99999999999998934, 194.7500000012290400, 15.58845726811991561 ) ) ;
#27100=CARTESIAN_POINT ( 'NONE',  ( -7.234628195640316228, 199.0075961894323200, -27.00000000000000000 ) ) ;
#27104=CARTESIAN_POINT ( 'NONE',  ( 27.24356964375000700, 195.5468750006145342, 15.72908226750537075 ) ) ;
#27115=CARTESIAN_POINT ( 'NONE',  ( 27.24356964375000700, 196.4468750006145399, 15.72908226750537075 ) ) ;
#27126=CARTESIAN_POINT ( 'NONE',  ( 13.62178482187501416, 195.9031250006145513, 23.59362340125806767 ) ) ;
#27151=CARTESIAN_POINT ( 'NONE',  ( 13.62178482187499640, 199.6531250006145228, -23.59362340125807123 ) ) ;
#27185=ORIENTED_EDGE ( 'NONE', *, *, #18939, .F. ) ;
#27187=CARTESIAN_POINT ( 'NONE',  ( -13.62178482187498396, 198.5281250006145228, 23.59362340125808188 ) ) ;
#27196=ORIENTED_EDGE ( 'NONE', *, *, #2732, .F. ) ;
#27203=CARTESIAN_POINT ( 'NONE',  ( 13.49999999999999645, 198.0500000000000114, -23.38268590217984766 ) ) ;
#27210=LINE ( 'NONE', #669, #14597 ) ;
#27213=CARTESIAN_POINT ( 'NONE',  ( -27.00000000000000355, 198.3125000012290400, 0.000000000000000000 ) ) ;
#27251=ORIENTED_EDGE ( 'NONE', *, *, #6200, .T. ) ;
#27279=CARTESIAN_POINT ( 'NONE',  ( -3.253724281355068545E-15, 197.6374999999999602, -27.00000000000000000 ) ) ;
#27288=ORIENTED_EDGE ( 'NONE', *, *, #24015, .F. ) ;
#27298=CARTESIAN_POINT ( 'NONE',  ( 27.24356964375000345, 196.0343750006145456, -3.336375036156643733E-15 ) ) ;
#27306=EDGE_CURVE ( 'NONE', #36429, #10880, #9293, .T. ) ;
#27311=CARTESIAN_POINT ( 'NONE',  ( 27.24356964374999635, 196.9156250006145399, -15.72908226750539029 ) ) ;
#27314=EDGE_CURVE ( 'NONE', #21721, #36429, #1761, .T. ) ;
#27324=CARTESIAN_POINT ( 'NONE',  ( 1.069080835302379631E-14, 198.3124999999999716, 27.00000000000000000 ) ) ;
#27337=CARTESIAN_POINT ( 'NONE',  ( -27.24356964374999990, 198.4156250006145399, -15.72908226750537786 ) ) ;
#27362=CARTESIAN_POINT ( 'NONE',  ( 7.234628195640269155, 195.7450961906613713, 27.00000000000003197 ) ) ;
#27373=CARTESIAN_POINT ( 'NONE',  ( 27.24356964375000700, 196.8406250006145228, 15.72908226750537075 ) ) ;
#27388=CARTESIAN_POINT ( 'NONE',  ( -13.49999999999998401, 196.4750000000000227, 23.38268590217985476 ) ) ;
#27431=ORIENTED_EDGE ( 'NONE', *, *, #26389, .F. ) ;
#27451=EDGE_CURVE ( 'NONE', #13180, #22009, #30652, .T. ) ;
#27472=CARTESIAN_POINT ( 'NONE',  ( 0.000000000000000000, 200.0000000000000000, -27.00000000000000355 ) ) ;
#27477=VERTEX_POINT ( 'NONE', #27324 ) ;
#27481=ADVANCED_FACE ( 'NONE', ( #1352 ), #27699, .T. ) ;
#27487=CARTESIAN_POINT ( 'NONE',  ( -13.62178482187500528, 196.6343750006145399, -23.59362340125807123 ) ) ;
#27491=( BOUNDED_CURVE ( )  B_SPLINE_CURVE ( 2, ( #19810, #31345, #37389, #2713, #16951, #25655, #11255, #34557, #22825 ),
 .UNSPECIFIED., .F., .F. ) 
 B_SPLINE_CURVE_WITH_KNOTS ( ( 3, 2, 2, 2, 3 ),
 ( 0.7291666666666667407, 0.7361111111111111605, 0.7500000000000000000, 0.7638888888888888395, 0.7708333333333333703 ),
 .UNSPECIFIED. ) 
 CURVE ( )  GEOMETRIC_REPRESENTATION_ITEM ( )  RATIONAL_B_SPLINE_CURVE ( ( 0.9330127018922192983, 0.9330127018922198534, 1.000000000000000000, 0.8660254037844387076, 1.000000000000000000, 0.8660254037844387076, 1.000000000000000000, 0.9330127018922187432, 0.9330127018922192983 ) ) 
 REPRESENTATION_ITEM ( '' )  );
#27504=CARTESIAN_POINT ( 'NONE',  ( 13.62178482187501416, 197.2531250006145456, 23.59362340125806767 ) ) ;
#27527=CARTESIAN_POINT ( 'NONE',  ( 27.24356964375000700, 198.6406250006145058, 15.72908226750537075 ) ) ;
#27557=CARTESIAN_POINT ( 'NONE',  ( -27.00000000000000355, 198.2000000000000171, 0.000000000000000000 ) ) ;
#27561=CARTESIAN_POINT ( 'NONE',  ( -3.253724281355068545E-15, 197.3000000012290229, -27.00000000000000000 ) ) ;
#27564=CARTESIAN_POINT ( 'NONE',  ( -13.62178482187500528, 196.5781250006145342, -23.59362340125807123 ) ) ;
#27566=CYLINDRICAL_SURFACE ( 'NONE', #7480, 27.00000000000000355 ) ;
#27568=CARTESIAN_POINT ( 'NONE',  ( 26.99999999999999645, 196.3250000012290570, -15.58845726811990495 ) ) ;
#27580=CARTESIAN_POINT ( 'NONE',  ( 5.727106289114498080E-15, 198.7625000000000455, 31.17691453623979214 ) ) ;
#27588=CARTESIAN_POINT ( 'NONE',  ( -27.00000000000000355, 196.4000000000000057, 0.000000000000000000 ) ) ;
#27606=CARTESIAN_POINT ( 'NONE',  ( -13.49999999999998401, 196.1375000012290286, 23.38268590217985476 ) ) ;
#27609=CARTESIAN_POINT ( 'NONE',  ( 0.000000000000000000, 200.0000000000000000, 0.000000000000000000 ) ) ;
#27658=CARTESIAN_POINT ( 'NONE',  ( -7.234628195640316228, 197.6575961894323257, -27.00000000000000000 ) ) ;
#27659=CARTESIAN_POINT ( 'NONE',  ( -7.234628195640354420, 195.7049038117966404, 26.99999999999996803 ) ) ;
#27673=( BOUNDED_CURVE ( )  B_SPLINE_CURVE ( 2, ( #22249, #30960, #4978, #16005, #16560, #28106, #1580, #27362, #2137 ),
 .UNSPECIFIED., .F., .F. ) 
 B_SPLINE_CURVE_WITH_KNOTS ( ( 3, 2, 2, 2, 3 ),
 ( 0.6875000000000000000, 0.6944444444444444198, 0.7083333333333333703, 0.7222222222222222099, 0.7291666666666667407 ),
 .UNSPECIFIED. ) 
 CURVE ( )  GEOMETRIC_REPRESENTATION_ITEM ( )  RATIONAL_B_SPLINE_CURVE ( ( 0.9330127018922194093, 0.9330127018922194093, 1.000000000000000000, 0.8660254037844387076, 1.000000000000000000, 0.8660254037844387076, 1.000000000000000000, 0.9330127018922187432, 0.9330127018922192983 ) ) 
 REPRESENTATION_ITEM ( '' )  );
#27675=CARTESIAN_POINT ( 'NONE',  ( -13.62178482187498396, 195.4343750006145228, 23.59362340125808188 ) ) ;
#27687=CARTESIAN_POINT ( 'NONE',  ( -13.62178482187498396, 195.8281250006145342, 23.59362340125808188 ) ) ;
#27699=CYLINDRICAL_SURFACE ( 'NONE', #28236, 27.00000000000000355 ) ;
#27707=DIRECTION ( 'NONE',  ( 0.000000000000000000, 0.000000000000000000, -1.000000000000000000 ) ) ;
#27711=CARTESIAN_POINT ( 'NONE',  ( 5.778771075727756162E-15, 197.2156250006145513, 31.45816453501075927 ) ) ;
#27714=FACE_OUTER_BOUND ( 'NONE', #15655, .T. ) ;
#27747=CARTESIAN_POINT ( 'NONE',  ( 3.306546357697854128E-15, 200.0000000000000000, 27.00000000000000355 ) ) ;
#27750=CARTESIAN_POINT ( 'NONE',  ( 27.24356964375000345, 195.9781250006145399, -3.336375036156643733E-15 ) ) ;
#27751=CARTESIAN_POINT ( 'NONE',  ( 27.24356964374999635, 197.4218750006145342, -15.72908226750539029 ) ) ;
#27766=CARTESIAN_POINT ( 'NONE',  ( -13.49999999999998401, 198.2750000000000057, 23.38268590217985476 ) ) ;
#27774=CARTESIAN_POINT ( 'NONE',  ( -13.50000000000000533, 196.3249999999999886, -23.38268590217984411 ) ) ;
#27782=( BOUNDED_CURVE ( )  B_SPLINE_CURVE ( 2, ( #16039, #7316, #19076, #36110, #27588, #1617, #27774, #13187, #24377 ),
 .UNSPECIFIED., .F., .F. ) 
 B_SPLINE_CURVE_WITH_KNOTS ( ( 3, 2, 2, 2, 3 ),
 ( 0.6458333333333333703, 0.6527777777777777901, 0.6666666666666666297, 0.6805555555555555802, 0.6875000000000000000 ),
 .UNSPECIFIED. ) 
 CURVE ( )  GEOMETRIC_REPRESENTATION_ITEM ( )  RATIONAL_B_SPLINE_CURVE ( ( 0.9330127018922192983, 0.9330127018922198534, 1.000000000000000000, 0.8660254037844387076, 1.000000000000000000, 0.8660254037844387076, 1.000000000000000000, 0.9330127018922194093, 0.9330127018922194093 ) ) 
 REPRESENTATION_ITEM ( '' )  );
#27809=DIRECTION ( 'NONE',  ( -0.000000000000000000, -1.000000000000000000, -0.000000000000000000 ) ) ;
#27857=CIRCLE ( 'NONE', #12103, 27.00000000000000355 ) ;
#27868=CARTESIAN_POINT ( 'NONE',  ( -27.00000000000000355, 198.7250000012290059, -15.58845726811989429 ) ) ;
#27872=( BOUNDED_CURVE ( )  B_SPLINE_CURVE ( 2, ( #23803, #17562, #11671, #35343, #29666, #14896, #32504, #9208, #15270 ),
 .UNSPECIFIED., .F., .F. ) 
 B_SPLINE_CURVE_WITH_KNOTS ( ( 3, 2, 2, 2, 3 ),
 ( 0.4375000000000000000, 0.4444444444444444198, 0.4583333333333333148, 0.4722222222222222099, 0.4791666666666666852 ),
 .UNSPECIFIED. ) 
 CURVE ( )  GEOMETRIC_REPRESENTATION_ITEM ( )  RATIONAL_B_SPLINE_CURVE ( ( 0.9330127018922194093, 0.9330127018922194093, 1.000000000000000000, 0.8660254037844387076, 1.000000000000000000, 0.8660254037844387076, 1.000000000000000000, 0.9330127018922190762, 0.9330127018922194093 ) ) 
 REPRESENTATION_ITEM ( '' )  );
#27880=CARTESIAN_POINT ( 'NONE',  ( 7.234628195640322446, 195.2950961906613827, 26.99999999999999645 ) ) ;
#27884=CARTESIAN_POINT ( 'NONE',  ( 13.50000000000001421, 197.9000000000000341, 23.38268590217984055 ) ) ;
#27893=CARTESIAN_POINT ( 'NONE',  ( 27.24356964375000345, 197.3281250006145342, -3.336375036156643733E-15 ) ) ;
#27908=UNCERTAINTY_MEASURE_WITH_UNIT (LENGTH_MEASURE( 1.000000000000000082E-05 ), #34024, 'distance_accuracy_value', 'NONE');
#27922=( BOUNDED_CURVE ( )  B_SPLINE_CURVE ( 2, ( #33988, #9102, #14089, #31154, #17644, #12123, #2337, #8032, #2145 ),
 .UNSPECIFIED., .F., .F. ) 
 B_SPLINE_CURVE_WITH_KNOTS ( ( 3, 2, 2, 2, 3 ),
 ( 0.8541666666666667407, 0.8611111111111111605, 0.8750000000000000000, 0.8888888888888888395, 0.8958333333333333703 ),
 .UNSPECIFIED. ) 
 CURVE ( )  GEOMETRIC_REPRESENTATION_ITEM ( )  RATIONAL_B_SPLINE_CURVE ( ( 0.9330127018922192983, 0.9330127018922198534, 1.000000000000000000, 0.8660254037844387076, 1.000000000000000000, 0.8660254037844387076, 1.000000000000000000, 0.9330127018922187432, 0.9330127018922192983 ) ) 
 REPRESENTATION_ITEM ( '' )  );
#27933=CARTESIAN_POINT ( 'NONE',  ( -27.24356964374999990, 199.3718750006145513, -15.72908226750537786 ) ) ;
#27949=CARTESIAN_POINT ( 'NONE',  ( 26.99999999999999645, 198.0125000000000455, -15.58845726811990495 ) ) ;
#27953=EDGE_LOOP ( 'NONE', ( #11360, #19114, #4620, #19421 ) ) ;
#27999=CYLINDRICAL_SURFACE ( 'NONE', #2804, 27.00000000000000355 ) ;
#28011=CARTESIAN_POINT ( 'NONE',  ( -7.234628195640307347, 199.4575961894323370, -27.00000000000000711 ) ) ;
#28045=CARTESIAN_POINT ( 'NONE',  ( -27.24356964374999279, 195.8468750006145740, 15.72908226750539384 ) ) ;
#28056=CARTESIAN_POINT ( 'NONE',  ( -27.00000000000000355, 198.2750000012290741, -15.58845726811989429 ) ) ;
#28067=CARTESIAN_POINT ( 'NONE',  ( 27.00000000000000355, 195.3875000012290286, -3.306546357697854128E-15 ) ) ;
#28070=CARTESIAN_POINT ( 'NONE',  ( 5.438367727407757144E-14, 198.0875000000000057, -27.00000000000000000 ) ) ;
#28078=CARTESIAN_POINT ( 'NONE',  ( 27.24356964375000700, 195.0406250006145399, 15.72908226750537075 ) ) ;
#28106=CARTESIAN_POINT ( 'NONE',  ( 27.00000000000001421, 195.8000000012290513, 15.58845726811988897 ) ) ;
#28113=EDGE_CURVE ( 'NONE', #5775, #4383, #5626, .T. ) ;
#28118=CARTESIAN_POINT ( 'NONE',  ( -27.24356964374999635, 197.6468750006145285, 15.72908226750539384 ) ) ;
#28121=CARTESIAN_POINT ( 'NONE',  ( 1.069080835302379631E-14, 195.6124999999999829, 27.00000000000000000 ) ) ;
#28135=CARTESIAN_POINT ( 'NONE',  ( -27.24356964375000345, 199.4093750006145456, 0.000000000000000000 ) ) ;
#28186=ADVANCED_FACE ( 'NONE', ( #12148 ), #10500, .F. ) ;
#28203=( BOUNDED_CURVE ( )  B_SPLINE_CURVE ( 2, ( #31585, #25898, #17006, #17380, #10941, #23064, #2957, #3144, #11675 ),
 .UNSPECIFIED., .F., .F. ) 
 B_SPLINE_CURVE_WITH_KNOTS ( ( 3, 2, 2, 2, 3 ),
 ( 0.5625000000000000000, 0.5694444444444444198, 0.5833333333333333703, 0.5972222222222222099, 0.6041666666666667407 ),
 .UNSPECIFIED. ) 
 CURVE ( )  GEOMETRIC_REPRESENTATION_ITEM ( )  RATIONAL_B_SPLINE_CURVE ( ( 0.9330127018922194093, 0.9330127018922194093, 1.000000000000000000, 0.8660254037844387076, 1.000000000000000000, 0.8660254037844387076, 1.000000000000000000, 0.9330127018922187432, 0.9330127018922192983 ) ) 
 REPRESENTATION_ITEM ( '' )  );
#28214=CARTESIAN_POINT ( 'NONE',  ( -27.00000000000000355, 195.5750000012290570, -15.58845726811989429 ) ) ;
#28234=ORIENTED_EDGE ( 'NONE', *, *, #32700, .F. ) ;
#28236=AXIS2_PLACEMENT_3D ( 'NONE', #12924, #4759, #24666 ) ;
#28244=CARTESIAN_POINT ( 'NONE',  ( -27.00000000000000355, 199.1750000012290513, -15.58845726811989429 ) ) ;
#28266=CARTESIAN_POINT ( 'NONE',  ( -1.926257025242585782E-15, 196.9906250006145569, -31.45816453501075927 ) ) ;
#28284=DIRECTION ( 'NONE',  ( -0.000000000000000000, -1.000000000000000000, -0.000000000000000000 ) ) ;
#28302=CARTESIAN_POINT ( 'NONE',  ( 27.24356964375000700, 195.9406250006145456, 15.72908226750537075 ) ) ;
#28303=CARTESIAN_POINT ( 'NONE',  ( 27.24356964375000345, 198.7343750006145626, -3.336375036156643733E-15 ) ) ;
#28318=CARTESIAN_POINT ( 'NONE',  ( -13.50000000000000533, 195.4250000000000114, -23.38268590217984411 ) ) ;
#28340=AXIS2_PLACEMENT_3D ( 'NONE', #5255, #302, #34437 ) ;
#28388=DIRECTION ( 'NONE',  ( -0.000000000000000000, -1.000000000000000000, -0.000000000000000000 ) ) ;
#28394=FACE_OUTER_BOUND ( 'NONE', #2090, .T. ) ;
#28418=CARTESIAN_POINT ( 'NONE',  ( 13.50000000000001421, 198.4625000012290172, 23.38268590217984055 ) ) ;
#28444=CARTESIAN_POINT ( 'NONE',  ( -27.24356964374999990, 195.2656250006145342, -15.72908226750537786 ) ) ;
#28452=VERTEX_POINT ( 'NONE', #16467 ) ;
#28459=EDGE_CURVE ( 'NONE', #15329, #26034, #13394, .T. ) ;
#28478=B_SPLINE_CURVE_WITH_KNOTS ( 'NONE', 3,
 ( #31849, #19941, #28627, #2665 ),
 .UNSPECIFIED., .F., .F.,
 ( 4, 4 ),
 ( 0.000000000000000000, 1.000000000000000000 ),
 .UNSPECIFIED. ) ;
#28483=CARTESIAN_POINT ( 'NONE',  ( -13.62178482187498396, 197.6843750006145228, 23.59362340125808188 ) ) ;
#28494=CARTESIAN_POINT ( 'NONE',  ( 27.00000000000001421, 197.1500000012290172, 15.58845726811988897 ) ) ;
#28500=CARTESIAN_POINT ( 'NONE',  ( -13.50000000000000533, 196.3249999999999886, -23.38268590217984411 ) ) ;
#28502=ORIENTED_EDGE ( 'NONE', *, *, #18466, .T. ) ;
#28523=CARTESIAN_POINT ( 'NONE',  ( 3.306546357697854128E-15, 200.0000000000000000, 27.00000000000000355 ) ) ;
#28550=ORIENTED_EDGE ( 'NONE', *, *, #1371, .F. ) ;
#28602=CARTESIAN_POINT ( 'NONE',  ( 26.99999999999999645, 197.6750000012290513, -15.58845726811990495 ) ) ;
#28627=CARTESIAN_POINT ( 'NONE',  ( -20.86978560514296532, 194.8401013911397683, -17.51182845191284798 ) ) ;
#28628=( BOUNDED_CURVE ( )  B_SPLINE_CURVE ( 2, ( #17832, #6630, #23888, #14975, #12314, #1124, #18391, #27100, #35429 ),
 .UNSPECIFIED., .F., .F. ) 
 B_SPLINE_CURVE_WITH_KNOTS ( ( 3, 2, 2, 2, 3 ),
 ( 0.1458333333333333426, 0.1527777777777777901, 0.1666666666666666574, 0.1805555555555555525, 0.1875000000000000000 ),
 .UNSPECIFIED. ) 
 CURVE ( )  GEOMETRIC_REPRESENTATION_ITEM ( )  RATIONAL_B_SPLINE_CURVE ( ( 0.9330127018922194093, 0.9330127018922194093, 1.000000000000000000, 0.8660254037844387076, 1.000000000000000000, 0.8660254037844387076, 1.000000000000000000, 0.9330127018922194093, 0.9330127018922194093 ) ) 
 REPRESENTATION_ITEM ( '' )  );
#28656=CARTESIAN_POINT ( 'NONE',  ( 1.120210788295102201E-13, 196.7375000000000398, -27.00000000000000711 ) ) ;
#28664=CARTESIAN_POINT ( 'NONE',  ( -27.00000000000000355, 198.7250000012290343, -15.58845726811989429 ) ) ;
#28665=CARTESIAN_POINT ( 'NONE',  ( 13.62178482187499640, 196.5593750006145513, -23.59362340125807123 ) ) ;
#28683=CARTESIAN_POINT ( 'NONE',  ( -13.62178482187500528, 199.7843750006145456, -23.59362340125807123 ) ) ;
#28684=ORIENTED_EDGE ( 'NONE', *, *, #23360, .F. ) ;
#28685=ORIENTED_EDGE ( 'NONE', *, *, #9132, .F. ) ;
#28766=CARTESIAN_POINT ( 'NONE',  ( 1.120210788295102201E-13, 197.1875000000000568, -27.00000000000000711 ) ) ;
#28789=CARTESIAN_POINT ( 'NONE',  ( 13.49999999999999645, 195.9125000012290343, -23.38268590217984766 ) ) ;
#28798=VECTOR ( 'NONE', #22030, 1000.000000000000000 ) ;
#28820=CARTESIAN_POINT ( 'NONE',  ( -27.24356964375000345, 198.4718750006145171, -15.72908226750537786 ) ) ;
#28831=CARTESIAN_POINT ( 'NONE',  ( 27.24356964374999635, 198.7156250006145513, -15.72908226750539029 ) ) ;
#28834=DIRECTION ( 'NONE',  ( 0.000000000000000000, 0.000000000000000000, -1.000000000000000000 ) ) ;
#28852=CARTESIAN_POINT ( 'NONE',  ( 7.234628195640363302, 195.3674038105676800, -26.99999999999996803 ) ) ;
#28854=CARTESIAN_POINT ( 'NONE',  ( -13.62178482187498396, 196.3343750006145285, 23.59362340125808188 ) ) ;
#28856=CARTESIAN_POINT ( 'NONE',  ( 5.438367727407757144E-14, 198.5374999999999943, -27.00000000000000000 ) ) ;
#28873=CARTESIAN_POINT ( 'NONE',  ( -26.99999999999998934, 195.5374999999999943, 15.58845726811991561 ) ) ;
#28875=ORIENTED_EDGE ( 'NONE', *, *, #15193, .F. ) ;
#28903=CARTESIAN_POINT ( 'NONE',  ( 13.62178482187499640, 199.2031250006145342, -23.59362340125807123 ) ) ;
#28932=ADVANCED_FACE ( 'NONE', ( #11874 ), #20798, .T. ) ;
#28943=ORIENTED_EDGE ( 'NONE', *, *, #37043, .T. ) ;
#28974=CARTESIAN_POINT ( 'NONE',  ( -27.00000000000000355, 195.5750000012290286, -15.58845726811989429 ) ) ;
#29002=CARTESIAN_POINT ( 'NONE',  ( -13.62178482187498396, 199.4843750006145626, 23.59362340125808188 ) ) ;
#29012=CARTESIAN_POINT ( 'NONE',  ( 13.62178482187499640, 199.6531250006145228, -23.59362340125807123 ) ) ;
#29019=EDGE_CURVE ( 'NONE', #5529, #32564, #872, .T. ) ;
#29021=ORIENTED_EDGE ( 'NONE', *, *, #7091, .F. ) ;
#29034=CARTESIAN_POINT ( 'NONE',  ( -27.24356964374999635, 195.3968750006145569, 15.72908226750539384 ) ) ;
#29045=EDGE_CURVE ( 'NONE', #5775, #2631, #27044, .T. ) ;
#29052=CARTESIAN_POINT ( 'NONE',  ( -1.926257025242585782E-15, 198.3968750006145285, -31.45816453501075927 ) ) ;
#29064=AXIS2_PLACEMENT_3D ( 'NONE', #33049, #15434, #12769 ) ;
#29083=CARTESIAN_POINT ( 'NONE',  ( -27.24356964375000345, 198.9031250006145228, 0.000000000000000000 ) ) ;
#29090=CARTESIAN_POINT ( 'NONE',  ( -13.49999999999998401, 197.9375000012290400, 23.38268590217985476 ) ) ;
#29137=LINE ( 'NONE', #896, #22120 ) ;
#29157=CARTESIAN_POINT ( 'NONE',  ( 5.727106289114498080E-15, 196.1750000012290513, 31.17691453623979214 ) ) ;
#29179=CARTESIAN_POINT ( 'NONE',  ( 27.24356964374999635, 195.1718750006145342, -15.72908226750539029 ) ) ;
#29191=CARTESIAN_POINT ( 'NONE',  ( -13.62178482187500528, 199.3343750006145569, -23.59362340125807123 ) ) ;
#29204=CARTESIAN_POINT ( 'NONE',  ( -27.24356964375000345, 198.9031250006145228, 0.000000000000000000 ) ) ;
#29226=CARTESIAN_POINT ( 'NONE',  ( 27.24356964374999635, 196.9718750006145456, -15.72908226750539029 ) ) ;
#29243=CARTESIAN_POINT ( 'NONE',  ( -27.24356964374999990, 198.0218750006145569, -15.72908226750537786 ) ) ;
#29244=ADVANCED_FACE ( 'NONE', ( #8570 ), #17294, .T. ) ;
#29259=EDGE_CURVE ( 'NONE', #9546, #11516, #31139, .T. ) ;
#29272=CARTESIAN_POINT ( 'NONE',  ( -13.62178482187498396, 198.9781250006145399, 23.59362340125808188 ) ) ;
#29316=ORIENTED_EDGE ( 'NONE', *, *, #34329, .F. ) ;
#29338=CARTESIAN_POINT ( 'NONE',  ( 13.49999999999999645, 196.7000000000000171, -23.38268590217984766 ) ) ;
#29352=CARTESIAN_POINT ( 'NONE',  ( 26.99999999999999645, 196.3250000012290570, -15.58845726811990495 ) ) ;
#29363=FACE_OUTER_BOUND ( 'NONE', #35497, .T. ) ;
#29372=CARTESIAN_POINT ( 'NONE',  ( -27.24356964375000345, 196.7093750006145569, 0.000000000000000000 ) ) ;
#29383=CARTESIAN_POINT ( 'NONE',  ( 13.50000000000001421, 198.3499999999999943, 23.38268590217984055 ) ) ;
#29385=CARTESIAN_POINT ( 'NONE',  ( 5.778771075727756162E-15, 199.0718750006145399, 31.45816453501076637 ) ) ;
#29398=CARTESIAN_POINT ( 'NONE',  ( -27.24356964374999635, 198.0406250006145399, 15.72908226750539384 ) ) ;
#29410=VERTEX_POINT ( 'NONE', #37359 ) ;
#29420=CARTESIAN_POINT ( 'NONE',  ( -26.99999999999999645, 198.8000000012290513, 15.58845726811991561 ) ) ;
#29422=CARTESIAN_POINT ( 'NONE',  ( 27.24356964374999635, 195.1718750006145342, -15.72908226750539029 ) ) ;
#29438=CARTESIAN_POINT ( 'NONE',  ( -13.62178482187498396, 197.6843750006145228, 23.59362340125808188 ) ) ;
#29464=VECTOR ( 'NONE', #12444, 1000.000000000000000 ) ;
#29465=CARTESIAN_POINT ( 'NONE',  ( -13.62178482187498396, 199.4281250006145569, 23.59362340125808188 ) ) ;
#29484=ORIENTED_EDGE ( 'NONE', *, *, #9132, .T. ) ;
#29496=DIRECTION ( 'NONE',  ( 1.000000000000000000, 0.000000000000000000, 0.000000000000000000 ) ) ;
#29547=CLOSED_SHELL ( 'NONE', ( #8091, #3941, #22800, #15207, #21428, #21752, #8564, #36028, #27481, #25810, #28932, #3386, #8941, #30685, #34180, #36449, #5715, #11344, #7413, #31595, #5182, #32376, #11296, #29244, #26940, #31005, #11792, #15982, #24521, #8955, #1791, #26877, #1242, #12964, #23491, #28186 ) ) ;
#29565=CARTESIAN_POINT ( 'NONE',  ( 13.62178482187499640, 195.6593750006145456, -23.59362340125807123 ) ) ;
#29576=CARTESIAN_POINT ( 'NONE',  ( 27.24356964375000345, 197.3843750006145399, -3.336375036156643733E-15 ) ) ;
#29587=CARTESIAN_POINT ( 'NONE',  ( 27.24356964375000700, 197.7406250006145285, 15.72908226750537075 ) ) ;
#29595=CARTESIAN_POINT ( 'NONE',  ( 27.00000000000001421, 197.0374999999999943, 15.58845726811988897 ) ) ;
#29612=CARTESIAN_POINT ( 'NONE',  ( -27.24356964375000345, 198.4531250006145342, 0.000000000000000000 ) ) ;
#29613=CARTESIAN_POINT ( 'NONE',  ( 1.069080835302379631E-14, 197.9750000012290343, 27.00000000000000000 ) ) ;
#29626=CARTESIAN_POINT ( 'NONE',  ( -13.62178482187498396, 197.2343750006145626, 23.59362340125808188 ) ) ;
#29646=DIRECTION ( 'NONE',  ( 0.7660444769304640689, 0.000000000000000000, 0.6427875693915772182 ) ) ;
#29655=FACE_OUTER_BOUND ( 'NONE', #14624, .T. ) ;
#29666=CARTESIAN_POINT ( 'NONE',  ( 27.00000000000000355, 197.5250000000000057, -3.306546357697854128E-15 ) ) ;
#29676=CARTESIAN_POINT ( 'NONE',  ( 1.120210788295102201E-13, 195.3875000000000455, -27.00000000000000711 ) ) ;
#29681=DIRECTION ( 'NONE',  ( -0.000000000000000000, -1.000000000000000000, -0.000000000000000000 ) ) ;
#29704=CARTESIAN_POINT ( 'NONE',  ( 1.120210788295102201E-13, 196.7375000000000398, -27.00000000000000711 ) ) ;
#29706=CARTESIAN_POINT ( 'NONE',  ( 13.49999999999999645, 199.8499999999999943, -23.38268590217984766 ) ) ;
#29748=CARTESIAN_POINT ( 'NONE',  ( 13.49999999999999645, 199.0625000012290400, -23.38268590217984766 ) ) ;
#29751=CARTESIAN_POINT ( 'NONE',  ( 13.62178482187501416, 196.4093750006145456, 23.59362340125806767 ) ) ;
#29762=CARTESIAN_POINT ( 'NONE',  ( 13.62178482187501416, 196.8593750006145342, 23.59362340125806767 ) ) ;
#29775=CARTESIAN_POINT ( 'NONE',  ( -27.24356964374999990, 195.7156250006145513, -15.72908226750537786 ) ) ;
#29784=CARTESIAN_POINT ( 'NONE',  ( 7.234628195640363302, 197.1674038105676914, -26.99999999999996803 ) ) ;
#29800=CARTESIAN_POINT ( 'NONE',  ( -13.62178482187500528, 197.9281250006145569, -23.59362340125807123 ) ) ;
#29804=EDGE_CURVE ( 'NONE', #32564, #32162, #6143, .T. ) ;
#29814=EDGE_LOOP ( 'NONE', ( #26129, #3449, #27288, #11587 ) ) ;
#29824=PLANE ( 'NONE',  #29064 ) ;
#29839=CARTESIAN_POINT ( 'NONE',  ( -27.24356964374999279, 197.5906250006144944, 15.72908226750539384 ) ) ;
#29840=DIRECTION ( 'NONE',  ( -0.000000000000000000, -1.000000000000000000, -0.000000000000000000 ) ) ;
#29855=( BOUNDED_CURVE ( )  B_SPLINE_CURVE ( 2, ( #22597, #21440, #12327, #23901, #3982, #20683, #29383, #948, #35443 ),
 .UNSPECIFIED., .F., .F. ) 
 B_SPLINE_CURVE_WITH_KNOTS ( ( 3, 2, 2, 2, 3 ),
 ( 0.2708333333333333703, 0.2777777777777777901, 0.2916666666666666852, 0.3055555555555555802, 0.3125000000000000000 ),
 .UNSPECIFIED. ) 
 CURVE ( )  GEOMETRIC_REPRESENTATION_ITEM ( )  RATIONAL_B_SPLINE_CURVE ( ( 0.9330127018922194093, 0.9330127018922196314, 1.000000000000000000, 0.8660254037844387076, 1.000000000000000000, 0.8660254037844387076, 1.000000000000000000, 0.9330127018922194093, 0.9330127018922194093 ) ) 
 REPRESENTATION_ITEM ( '' )  );
#29856=CARTESIAN_POINT ( 'NONE',  ( 5.438367727407757775E-14, 197.7500000012290400, -27.00000000000000355 ) ) ;
#29866=CARTESIAN_POINT ( 'NONE',  ( 1.069080835302379631E-14, 195.2750000012290457, 27.00000000000000000 ) ) ;
#29922=( BOUNDED_CURVE ( )  B_SPLINE_CURVE ( 2, ( #33629, #30788, #4811, #16391, #8589, #26578, #14281 ),
 .UNSPECIFIED., .F., .F. ) 
 B_SPLINE_CURVE_WITH_KNOTS ( ( 3, 2, 2, 3 ),
 ( 0.8958333333333333703, 0.9027777777777777901, 0.9166666666666666297, 0.9258785565094815873 ),
 .UNSPECIFIED. ) 
 CURVE ( )  GEOMETRIC_REPRESENTATION_ITEM ( )  RATIONAL_B_SPLINE_CURVE ( ( 0.9330127018922192983, 0.9330127018922198534, 1.000000000000000000, 0.8660254037844387076, 1.000000000000000000, 0.9111405360107182050, 0.9401542295229976531 ) ) 
 REPRESENTATION_ITEM ( '' )  );
#29945=CARTESIAN_POINT ( 'NONE',  ( -13.62178482187498396, 196.7843750006145456, 23.59362340125808188 ) ) ;
#29956=CARTESIAN_POINT ( 'NONE',  ( -13.62178482187500528, 197.5343750006145456, -23.59362340125807123 ) ) ;
#29967=CARTESIAN_POINT ( 'NONE',  ( -13.62178482187498396, 195.3781250006145171, 23.59362340125808188 ) ) ;
#29992=CARTESIAN_POINT ( 'NONE',  ( -27.24356964374999990, 199.3156250006145171, -15.72908226750537786 ) ) ;
#29993=FACE_OUTER_BOUND ( 'NONE', #26381, .T. ) ;
#30031=CARTESIAN_POINT ( 'NONE',  ( -27.24356964374999279, 198.4906250006145569, 15.72908226750539384 ) ) ;
#30032=CARTESIAN_POINT ( 'NONE',  ( 27.24356964375000345, 199.6343750006145399, -3.336375036156643733E-15 ) ) ;
#30048=CARTESIAN_POINT ( 'NONE',  ( -26.99999999999998934, 199.5874999999999773, 15.58845726811991561 ) ) ;
#30124=CARTESIAN_POINT ( 'NONE',  ( -3.253724281355068545E-15, 196.2874999999999659, -27.00000000000000000 ) ) ;
#30147=CARTESIAN_POINT ( 'NONE',  ( 13.62178482187499640, 197.4593750006145285, -23.59362340125807123 ) ) ;
#30159=CARTESIAN_POINT ( 'NONE',  ( -27.24356964375000345, 195.3031250006145285, 0.000000000000000000 ) ) ;
#30165=CARTESIAN_POINT ( 'NONE',  ( 0.000000000000000000, 200.0000000000000000, -27.00000000000000355 ) ) ;
#30170=CARTESIAN_POINT ( 'NONE',  ( -7.234628195640263826, 195.0700961906613600, -27.00000000000003553 ) ) ;
#30184=CARTESIAN_POINT ( 'NONE',  ( 13.62178482187499640, 198.7531250006145456, -23.59362340125807123 ) ) ;
#30223=CARTESIAN_POINT ( 'NONE',  ( 27.24356964375000345, 198.2281250006145399, -3.336375036156643733E-15 ) ) ;
#30225=CARTESIAN_POINT ( 'NONE',  ( 13.62178482187501416, 199.5593750006145513, 23.59362340125806767 ) ) ;
#30239=CARTESIAN_POINT ( 'NONE',  ( -26.99999999999998934, 197.7875000000000227, 15.58845726811991561 ) ) ;
#30267=EDGE_LOOP ( 'NONE', ( #14482, #9425, #32659, #3575 ) ) ;
#30280=FACE_OUTER_BOUND ( 'NONE', #26004, .T. ) ;
#30303=CARTESIAN_POINT ( 'NONE',  ( -26.99999999999998934, 195.2000000012290286, 15.58845726811991561 ) ) ;
#30310=( BOUNDED_SURFACE ( )  B_SPLINE_SURFACE ( 1, 2, ( 
 ( #35898, #15258, #9941, #21335, #6921, #18492, #30032, #21521, #30225, #19055, #8036, #31335, #4623, #27933, #36830, #7851, #13730, #5363, #22074, #2341, #19424, #4991, #25278, #33814, #33626, #5179, #25463, #10872, #31158, #19799, #28303, #37015, #13534, #13348, #14093, #13912, #11058, #22445, #30974, #16941, #33992, #24904, #30785, #16573, #25645, #4808, #19611, #16388, #7666, #25089, #16755, #22633, #34181, #1963, #8225, #36645, #10683, #36455, #28483, #28118, #19244, #2526, #37199, #11243, #2149, #27751, #22815, #22262, #34363, #30606, #10495, #16202, #1781, #34918, #26386, #8962, #11986, #29226, #8586, #5732, #5919, #31704, #17877, #25830, #23368, #20534, #9151, #14840, #28665, #20348, #17311, #2888, #20155, #17129, #28854, #31518, #6105, #34731, #32077, #14460, #2702, #26016, #17499, #37377, #44, #11610, #11429, #22997, #23184, #17688, #34546, #6306, #8775, #604, #3268, #420, #23558, #31890, #35103, #29034, #3078, #14278, #20718, #14647, #26197, #29422, #32262, #3456, #235, #11799, #15025, #26575, #12173, #23747, #8408 ),
 ( #19976, #5543, #1174, #1552, #27151, #10091, #35858, #24501, #7074, #35670, #32452, #21483, #24127, #29992, #26955, #6685, #18642, #9899, #12748, #15977, #24315, #35481, #4023, #33023, #23938, #1367, #18070, #26766, #30184, #4210, #6496, #27527, #30374, #15788, #9720, #13124, #29612, #27337, #15217, #12938, #21294, #6875, #32830, #36047, #35285, #9343, #21661, #33214, #3648, #7254, #29800, #18450, #20913, #15595, #21105, #18828, #798, #4395, #12368, #9530, #32643, #18256, #3833, #15411, #985, #12561, #27893, #19011, #34139, #27711, #19201, #25423, #4586, #13491, #1740, #28266, #24678, #19568, #36788, #13307, #21848, #10831, #13874, #10643, #22406, #13689, #8186, #33953, #31298, #11019, #7996, #16162, #36976, #22221, #31120, #5138, #4949, #16719, #30932, #30569, #24866, #36414, #10273, #2298, #25049, #22593, #30748, #7439, #33586, #33773, #10457, #7626, #22035, #4771, #16344, #1923, #19761, #36602, #5327, #7813, #16903, #28444, #19389, #33400, #2482, #36232, #16531, #28078, #2111, #25237, #8370, #20308, #3039, #25975, #34324 ) ),
 .UNSPECIFIED., .F., .F., .F. ) 
 B_SPLINE_SURFACE_WITH_KNOTS ( ( 2, 2 ),
 ( 3, 2, 2, 2, 2, 2, 2, 2, 2, 2, 2, 2, 2, 2, 2, 2, 2, 2, 2, 2, 2, 2, 2, 2, 2, 2, 2, 2, 2, 2, 2, 2, 2, 2, 2, 2, 2, 2, 2, 2, 2, 2, 2, 2, 2, 2, 2, 2, 2, 2, 2, 2, 2, 2, 2, 2, 2, 2, 2, 2, 2, 2, 2, 2, 2, 2, 2, 3 ),
 ( 0.000000000000000000, 1.000000000000000000 ),
 ( 0.000000000000000000, 0.01388888888888888812, 0.02777777777777777624, 0.04166666666666666435, 0.05555555555555555247, 0.06944444444444444753, 0.08333333333333332871, 0.09722222222222222376, 0.1111111111111111049, 0.1250000000000000000, 0.1388888888888888951, 0.1527777777777777901, 0.1666666666666666574, 0.1805555555555555525, 0.1944444444444444475, 0.2083333333333333426, 0.2222222222222222099, 0.2361111111111111049, 0.2500000000000000000, 0.2638888888888888951, 0.2777777777777777901, 0.2916666666666666852, 0.3055555555555555802, 0.3194444444444444198, 0.3333333333333333148, 0.3472222222222222099, 0.3611111111111111049, 0.3750000000000000000, 0.3888888888888888951, 0.4027777777777777901, 0.4166666666666666852, 0.4305555555555555802, 0.4444444444444444198, 0.4583333333333333148, 0.4722222222222222099, 0.4861111111111111049, 0.5000000000000000000, 0.5138888888888888395, 0.5277777777777777901, 0.5416666666666666297, 0.5555555555555555802, 0.5694444444444444198, 0.5833333333333333703, 0.5972222222222222099, 0.6111111111111111605, 0.6250000000000000000, 0.6388888888888888395, 0.6527777777777777901, 0.6666666666666666297, 0.6805555555555555802, 0.6944444444444444198, 0.7083333333333333703, 0.7222222222222222099, 0.7361111111111111605, 0.7500000000000000000, 0.7638888888888888395, 0.7777777777777777901, 0.7916666666666666297, 0.8055555555555555802, 0.8194444444444444198, 0.8333333333333333703, 0.8472222222222222099, 0.8611111111111111605, 0.8750000000000000000, 0.8888888888888888395, 0.9027777777777777901, 0.9166666666666666297, 0.9258785558287927486 ),
 .UNSPECIFIED. ) 
 GEOMETRIC_REPRESENTATION_ITEM ( )  RATIONAL_B_SPLINE_SURFACE ( (
 ( 1.000000000000000000, 0.8660254037844387076, 1.000000000000000000, 0.8660254037844387076, 1.000000000000000000, 0.8660254037844387076, 1.000000000000000000, 0.8660254037844387076, 1.000000000000000000, 0.8660254037844387076, 1.000000000000000000, 0.8660254037844387076, 1.000000000000000000, 0.8660254037844387076, 1.000000000000000000, 0.8660254037844387076, 1.000000000000000000, 0.8660254037844387076, 1.000000000000000000, 0.8660254037844387076, 1.000000000000000000, 0.8660254037844387076, 1.000000000000000000, 0.8660254037844387076, 1.000000000000000000, 0.8660254037844387076, 1.000000000000000000, 0.8660254037844387076, 1.000000000000000000, 0.8660254037844387076, 1.000000000000000000, 0.8660254037844387076, 1.000000000000000000, 0.8660254037844387076, 1.000000000000000000, 0.8660254037844387076, 1.000000000000000000, 0.8660254037844387076, 1.000000000000000000, 0.8660254037844387076, 1.000000000000000000, 0.8660254037844387076, 1.000000000000000000, 0.8660254037844387076, 1.000000000000000000, 0.8660254037844387076, 1.000000000000000000, 0.8660254037844387076, 1.000000000000000000, 0.8660254037844387076, 1.000000000000000000, 0.8660254037844387076, 1.000000000000000000, 0.8660254037844387076, 1.000000000000000000, 0.8660254037844387076, 1.000000000000000000, 0.8660254037844387076, 1.000000000000000000, 0.8660254037844387076, 1.000000000000000000, 0.8660254037844387076, 1.000000000000000000, 0.8660254037844387076, 1.000000000000000000, 0.8660254037844387076, 1.000000000000000000, 0.8660254037844387076, 1.000000000000000000, 0.8660254037844387076, 1.000000000000000000, 0.8660254037844387076, 1.000000000000000000, 0.8660254037844387076, 1.000000000000000000, 0.8660254037844387076, 1.000000000000000000, 0.8660254037844387076, 1.000000000000000000, 0.8660254037844387076, 1.000000000000000000, 0.8660254037844387076, 1.000000000000000000, 0.8660254037844387076, 1.000000000000000000, 0.8660254037844387076, 1.000000000000000000, 0.8660254037844387076, 1.000000000000000000, 0.8660254037844387076, 1.000000000000000000, 0.8660254037844387076, 1.000000000000000000, 0.8660254037844387076, 1.000000000000000000, 0.8660254037844387076, 1.000000000000000000, 0.8660254037844387076, 1.000000000000000000, 0.8660254037844387076, 1.000000000000000000, 0.8660254037844387076, 1.000000000000000000, 0.8660254037844387076, 1.000000000000000000, 0.8660254037844387076, 1.000000000000000000, 0.8660254037844387076, 1.000000000000000000, 0.8660254037844387076, 1.000000000000000000, 0.8660254037844387076, 1.000000000000000000, 0.8660254037844387076, 1.000000000000000000, 0.8660254037844387076, 1.000000000000000000, 0.8660254037844387076, 1.000000000000000000, 0.8660254037844387076, 1.000000000000000000, 0.8660254037844387076, 1.000000000000000000, 0.8660254037844387076, 1.000000000000000000, 0.8660254037844387076, 1.000000000000000000, 0.8660254037844387076, 1.000000000000000000, 0.8660254037844387076, 1.000000000000000000, 0.8660254037844387076, 1.000000000000000000, 0.9111405425767590271, 0.9401542252352144136),
 ( 1.000000000000000000, 0.8660254037844387076, 1.000000000000000000, 0.8660254037844387076, 1.000000000000000000, 0.8660254037844387076, 1.000000000000000000, 0.8660254037844387076, 1.000000000000000000, 0.8660254037844387076, 1.000000000000000000, 0.8660254037844387076, 1.000000000000000000, 0.8660254037844387076, 1.000000000000000000, 0.8660254037844387076, 1.000000000000000000, 0.8660254037844387076, 1.000000000000000000, 0.8660254037844387076, 1.000000000000000000, 0.8660254037844387076, 1.000000000000000000, 0.8660254037844387076, 1.000000000000000000, 0.8660254037844387076, 1.000000000000000000, 0.8660254037844387076, 1.000000000000000000, 0.8660254037844387076, 1.000000000000000000, 0.8660254037844387076, 1.000000000000000000, 0.8660254037844387076, 1.000000000000000000, 0.8660254037844387076, 1.000000000000000000, 0.8660254037844387076, 1.000000000000000000, 0.8660254037844387076, 1.000000000000000000, 0.8660254037844387076, 1.000000000000000000, 0.8660254037844387076, 1.000000000000000000, 0.8660254037844387076, 1.000000000000000000, 0.8660254037844387076, 1.000000000000000000, 0.8660254037844387076, 1.000000000000000000, 0.8660254037844387076, 1.000000000000000000, 0.8660254037844387076, 1.000000000000000000, 0.8660254037844387076, 1.000000000000000000, 0.8660254037844387076, 1.000000000000000000, 0.8660254037844387076, 1.000000000000000000, 0.8660254037844387076, 1.000000000000000000, 0.8660254037844387076, 1.000000000000000000, 0.8660254037844387076, 1.000000000000000000, 0.8660254037844387076, 1.000000000000000000, 0.8660254037844387076, 1.000000000000000000, 0.8660254037844387076, 1.000000000000000000, 0.8660254037844387076, 1.000000000000000000, 0.8660254037844387076, 1.000000000000000000, 0.8660254037844387076, 1.000000000000000000, 0.8660254037844387076, 1.000000000000000000, 0.8660254037844387076, 1.000000000000000000, 0.8660254037844387076, 1.000000000000000000, 0.8660254037844387076, 1.000000000000000000, 0.8660254037844387076, 1.000000000000000000, 0.8660254037844387076, 1.000000000000000000, 0.8660254037844387076, 1.000000000000000000, 0.8660254037844387076, 1.000000000000000000, 0.8660254037844387076, 1.000000000000000000, 0.8660254037844387076, 1.000000000000000000, 0.8660254037844387076, 1.000000000000000000, 0.8660254037844387076, 1.000000000000000000, 0.8660254037844387076, 1.000000000000000000, 0.8660254037844387076, 1.000000000000000000, 0.8660254037844387076, 1.000000000000000000, 0.8660254037844387076, 1.000000000000000000, 0.8660254037844387076, 1.000000000000000000, 0.8660254037844387076, 1.000000000000000000, 0.8660254037844387076, 1.000000000000000000, 0.8660254037844387076, 1.000000000000000000, 0.8660254037844387076, 1.000000000000000000, 0.8660254037844387076, 1.000000000000000000, 0.8660254037844387076, 1.000000000000000000, 0.8660254037844387076, 1.000000000000000000, 0.8660254037844387076, 1.000000000000000000, 0.8660254037844387076, 1.000000000000000000, 0.8660254037844387076, 1.000000000000000000, 0.9111405425767590271, 0.9401542252352144136) ) ) 
 REPRESENTATION_ITEM ( '' )  SURFACE ( )  );
#30316=CARTESIAN_POINT ( 'NONE',  ( -27.00000000000000355, 197.7500000000000000, 0.000000000000000000 ) ) ;
#30335=CARTESIAN_POINT ( 'NONE',  ( 5.778771075727756162E-15, 197.7218750006145456, 31.45816453501076637 ) ) ;
#30348=CARTESIAN_POINT ( 'NONE',  ( 27.24356964375000700, 197.2906250006145399, 15.72908226750537075 ) ) ;
#30355=DIRECTION ( 'NONE',  ( -0.000000000000000000, -1.000000000000000000, -0.000000000000000000 ) ) ;
#30374=CARTESIAN_POINT ( 'NONE',  ( 13.62178482187501416, 198.6031250006145399, 23.59362340125806767 ) ) ;
#30412=CARTESIAN_POINT ( 'NONE',  ( 27.24356964374999279, 196.9156250006145399, -15.72908226750539207 ) ) ;
#30431=CARTESIAN_POINT ( 'NONE',  ( -27.00000000000000355, 197.7125000000000057, -15.58845726811989429 ) ) ;
#30449=( NAMED_UNIT ( * ) PLANE_ANGLE_UNIT ( ) SI_UNIT ( $, .RADIAN. ) );
#30450=CARTESIAN_POINT ( 'NONE',  ( 3.306546357697854128E-15, 200.0000000000000000, 27.00000000000000355 ) ) ;
#30512=CARTESIAN_POINT ( 'NONE',  ( 1.120210788295102201E-13, 196.8500000012290343, -27.00000000000000711 ) ) ;
#30518=ORIENTED_EDGE ( 'NONE', *, *, #26598, .F. ) ;
#30534=CIRCLE ( 'NONE', #15318, 25.00000000000000000 ) ;
#30543=CARTESIAN_POINT ( 'NONE',  ( -27.24356964374999990, 196.1656250006145399, -15.72908226750537786 ) ) ;
#30555=CARTESIAN_POINT ( 'NONE',  ( -27.00000000000000355, 195.1625000012290343, 0.000000000000000000 ) ) ;
#30569=CARTESIAN_POINT ( 'NONE',  ( -1.926257025242585782E-15, 196.0906250006145228, -31.45816453501075927 ) ) ;
#30605=CARTESIAN_POINT ( 'NONE',  ( 27.24356964375000345, 196.8781250006145171, -3.336375036156643733E-15 ) ) ;
#30606=CARTESIAN_POINT ( 'NONE',  ( 5.778771075727756162E-15, 197.2718750006145569, 31.45816453501075927 ) ) ;
#30615=( NAMED_UNIT ( * ) SI_UNIT ( $, .STERADIAN. ) SOLID_ANGLE_UNIT ( ) );
#30620=CARTESIAN_POINT ( 'NONE',  ( -13.49999999999998401, 198.7250000000000227, 23.38268590217985476 ) ) ;
#30645=( BOUNDED_CURVE ( )  B_SPLINE_CURVE ( 2, ( #6304, #17875, #23183, #29420, #20154, #28664, #2701, #3454, #5731 ),
 .UNSPECIFIED., .F., .F. ) 
 B_SPLINE_CURVE_WITH_KNOTS ( ( 3, 2, 2, 2, 3 ),
 ( 0.1458333333333333426, 0.1527777777777777901, 0.1666666666666666574, 0.1805555555555555525, 0.1875000000000000000 ),
 .UNSPECIFIED. ) 
 CURVE ( )  GEOMETRIC_REPRESENTATION_ITEM ( )  RATIONAL_B_SPLINE_CURVE ( ( 0.9330127018922194093, 0.9330127018922194093, 1.000000000000000000, 0.8660254037844387076, 1.000000000000000000, 0.8660254037844387076, 1.000000000000000000, 0.9330127018922194093, 0.9330127018922194093 ) ) 
 REPRESENTATION_ITEM ( '' )  );
#30652=CIRCLE ( 'NONE', #19168, 5.000000000000000000 ) ;
#30685=ADVANCED_FACE ( 'NONE', ( #36387 ), #7783, .T. ) ;
#30714=CARTESIAN_POINT ( 'NONE',  ( 27.24356964375000345, 195.5843750006145285, -3.336375036156643733E-15 ) ) ;
#30725=CARTESIAN_POINT ( 'NONE',  ( 13.49999999999999645, 199.5125000012290286, -23.38268590217984766 ) ) ;
#30748=CARTESIAN_POINT ( 'NONE',  ( -13.62178482187498396, 195.8281250006145342, 23.59362340125808188 ) ) ;
#30784=CARTESIAN_POINT ( 'NONE',  ( -27.24356964375000345, 195.7156250006145513, -15.72908226750537786 ) ) ;
#30785=CARTESIAN_POINT ( 'NONE',  ( 27.24356964375000345, 198.2843750006145456, -3.336375036156643733E-15 ) ) ;
#30788=CARTESIAN_POINT ( 'NONE',  ( -7.234628195640354420, 195.1424038105676573, 26.99999999999996803 ) ) ;
#30793=ORIENTED_EDGE ( 'NONE', *, *, #20591, .F. ) ;
#30799=CARTESIAN_POINT ( 'NONE',  ( 26.99999999999999645, 197.1125000000000398, -15.58845726811990495 ) ) ;
#30803=AXIS2_PLACEMENT_3D ( 'NONE', #20064, #17032, #10960 ) ;
#30841=CARTESIAN_POINT ( 'NONE',  ( 5.438367727407757144E-14, 197.7500000012290400, -27.00000000000000000 ) ) ;
#30862=CARTESIAN_POINT ( 'NONE',  ( 1.069080835302379631E-14, 199.6625000000000227, 27.00000000000000000 ) ) ;
#30865=( BOUNDED_CURVE ( )  B_SPLINE_CURVE ( 2, ( #28070, #13865, #1731, #10825, #8178, #16336, #27884, #22026, #13683 ),
 .UNSPECIFIED., .F., .F. ) 
 B_SPLINE_CURVE_WITH_KNOTS ( ( 3, 2, 2, 2, 3 ),
 ( 0.3541666666666666852, 0.3611111111111111049, 0.3750000000000000000, 0.3888888888888888951, 0.3958333333333333703 ),
 .UNSPECIFIED. ) 
 CURVE ( )  GEOMETRIC_REPRESENTATION_ITEM ( )  RATIONAL_B_SPLINE_CURVE ( ( 0.9330127018922194093, 0.9330127018922196314, 1.000000000000000000, 0.8660254037844387076, 1.000000000000000000, 0.8660254037844387076, 1.000000000000000000, 0.9330127018922190762, 0.9330127018922194093 ) ) 
 REPRESENTATION_ITEM ( '' )  );
#30882=FACE_OUTER_BOUND ( 'NONE', #1665, .T. ) ;
#30894=CARTESIAN_POINT ( 'NONE',  ( -13.62178482187498396, 194.9843750006145626, 23.59362340125808188 ) ) ;
#30897=ORIENTED_EDGE ( 'NONE', *, *, #17818, .T. ) ;
#30906=CARTESIAN_POINT ( 'NONE',  ( 27.00000000000000355, 198.5375000012290627, -3.306546357697854128E-15 ) ) ;
#30918=ORIENTED_EDGE ( 'NONE', *, *, #28459, .F. ) ;
#30924=CARTESIAN_POINT ( 'NONE',  ( 26.99999999999999645, 199.3625000000000114, -15.58845726811990495 ) ) ;
#30932=CARTESIAN_POINT ( 'NONE',  ( -13.62178482187500528, 196.1281250006145171, -23.59362340125807123 ) ) ;
#30960=CARTESIAN_POINT ( 'NONE',  ( 7.234628195640309123, 195.9299038117966916, -27.00000000000000711 ) ) ;
#30973=CARTESIAN_POINT ( 'NONE',  ( -27.24356964375000345, 195.2656250006145342, -15.72908226750537786 ) ) ;
#30974=CARTESIAN_POINT ( 'NONE',  ( -13.62178482187500528, 198.4343750006145228, -23.59362340125807123 ) ) ;
#30991=CARTESIAN_POINT ( 'NONE',  ( 27.00000000000001066, 198.3875000000000171, 15.58845726811988897 ) ) ;
#31005=ADVANCED_FACE ( 'NONE', ( #30882 ), #24999, .T. ) ;
#31083=CARTESIAN_POINT ( 'NONE',  ( -20.86978606573367045, 194.8588513912095266, -17.51182790300216752 ) ) ;
#31095=CARTESIAN_POINT ( 'NONE',  ( 27.00000000000001066, 198.5000000012290400, 15.58845726811988897 ) ) ;
#31098=VECTOR ( 'NONE', #17977, 1000.000000000000000 ) ;
#31120=CARTESIAN_POINT ( 'NONE',  ( -13.62178482187498396, 196.2781250006145228, 23.59362340125808188 ) ) ;
#31139=LINE ( 'NONE', #30450, #23442 ) ;
#31144=EDGE_CURVE ( 'NONE', #20323, #24000, #23287, .T. ) ;
#31154=CARTESIAN_POINT ( 'NONE',  ( 26.99999999999999645, 194.9750000012290343, -15.58845726811990495 ) ) ;
#31155=ORIENTED_EDGE ( 'NONE', *, *, #19573, .T. ) ;
#31158=CARTESIAN_POINT ( 'NONE',  ( 13.62178482187499640, 198.8093750006145513, -23.59362340125807123 ) ) ;
#31175=CARTESIAN_POINT ( 'NONE',  ( -27.24356964375000345, 198.9593750006145285, 0.000000000000000000 ) ) ;
#31209=DIRECTION ( 'NONE',  ( 0.000000000000000000, 0.000000000000000000, -1.000000000000000000 ) ) ;
#31242=EDGE_CURVE ( 'NONE', #20323, #37392, #37176, .T. ) ;
#31246=CARTESIAN_POINT ( 'NONE',  ( -27.00000000000000355, 199.8312500006145171, 0.000000000000000000 ) ) ;
#31247=CARTESIAN_POINT ( 'NONE',  ( -27.24356964375000345, 199.3156250006145171, -15.72908226750537786 ) ) ;
#31276=CARTESIAN_POINT ( 'NONE',  ( -13.49999999999998401, 199.2875000012290627, 23.38268590217985476 ) ) ;
#31298=CARTESIAN_POINT ( 'NONE',  ( 13.62178482187499640, 196.5031250006145456, -23.59362340125807123 ) ) ;
#31312=ORIENTED_EDGE ( 'NONE', *, *, #2314, .T. ) ;
#31335=CARTESIAN_POINT ( 'NONE',  ( -27.24356964374999635, 199.4468750006145399, 15.72908226750539384 ) ) ;
#31345=CARTESIAN_POINT ( 'NONE',  ( -7.234628195640354420, 196.0424038105676630, 26.99999999999996803 ) ) ;
#31351=CARTESIAN_POINT ( 'NONE',  ( -1.926257025242585782E-15, 199.2968750006145342, -31.45816453501075927 ) ) ;
#31379=ORIENTED_EDGE ( 'NONE', *, *, #20765, .T. ) ;
#31428=FACE_OUTER_BOUND ( 'NONE', #20144, .T. ) ;
#31457=CARTESIAN_POINT ( 'NONE',  ( -26.99999999999998934, 198.3500000012290627, 15.58845726811991561 ) ) ;
#31490=AXIS2_PLACEMENT_3D ( 'NONE', #759, #9491, #23710 ) ;
#31496=EDGE_LOOP ( 'NONE', ( #33909, #18318, #4452, #28684 ) ) ;
#31517=CARTESIAN_POINT ( 'NONE',  ( -27.24356964374999279, 195.3406250006145228, 15.72908226750539384 ) ) ;
#31518=CARTESIAN_POINT ( 'NONE',  ( -27.24356964374999635, 196.2968750006145342, 15.72908226750539384 ) ) ;
#31536=CARTESIAN_POINT ( 'NONE',  ( 27.24356964375000700, 199.5968750006145456, 15.72908226750537075 ) ) ;
#31566=EDGE_CURVE ( 'NONE', #18034, #10170, #24036, .T. ) ;
#31585=CARTESIAN_POINT ( 'NONE',  ( 1.069080835302379631E-14, 196.6250000012290400, 27.00000000000000000 ) ) ;
#31595=ADVANCED_FACE ( 'NONE', ( #30280 ), #35581, .T. ) ;
#31608=EDGE_CURVE ( 'NONE', #32409, #34685, #11505, .T. ) ;
#31613=CARTESIAN_POINT ( 'NONE',  ( -7.234628195640263826, 196.8700961906613713, -27.00000000000003553 ) ) ;
#31615=CARTESIAN_POINT ( 'NONE',  ( 3.306546357697854128E-15, 200.0000000000000000, 27.00000000000000355 ) ) ;
#31640=CARTESIAN_POINT ( 'NONE',  ( 13.49999999999999645, 196.8125000012290400, -23.38268590217984766 ) ) ;
#31646=CIRCLE ( 'NONE', #25675, 5.000000000000000000 ) ;
#31670=CARTESIAN_POINT ( 'NONE',  ( -13.62178482187498396, 199.0343750006145456, 23.59362340125808188 ) ) ;
#31678=ORIENTED_EDGE ( 'NONE', *, *, #3211, .F. ) ;
#31680=CARTESIAN_POINT ( 'NONE',  ( -13.62178482187498396, 198.5281250006145228, 23.59362340125808188 ) ) ;
#31691=DIRECTION ( 'NONE',  ( 0.000000000000000000, 0.000000000000000000, 1.000000000000000000 ) ) ;
#31704=CARTESIAN_POINT ( 'NONE',  ( 5.778771075727756162E-15, 196.8218750006145399, 31.45816453501075927 ) ) ;
#31723=CARTESIAN_POINT ( 'NONE',  ( 5.778771075727756162E-15, 199.0718750006145399, 31.45816453501075927 ) ) ;
#31815=ORIENTED_EDGE ( 'NONE', *, *, #18426, .T. ) ;
#31823=CARTESIAN_POINT ( 'NONE',  ( -13.50000000000000533, 195.9875000012290229, -23.38268590217984411 ) ) ;
#31841=CARTESIAN_POINT ( 'NONE',  ( 13.49999999999999645, 196.8125000012290400, -23.38268590217984766 ) ) ;
#31849=CARTESIAN_POINT ( 'NONE',  ( -20.86978604919638869, 194.8026013911397456, -17.51182792271053046 ) ) ;
#31865=CARTESIAN_POINT ( 'NONE',  ( -13.62178482187500528, 198.3781250006145171, -23.59362340125807123 ) ) ;
#31890=CARTESIAN_POINT ( 'NONE',  ( 5.778771075727756162E-15, 195.4718750006145456, 31.45816453501075927 ) ) ;
#31892=CARTESIAN_POINT ( 'NONE',  ( -26.99999999999999645, 198.6875000000000284, 15.58845726811991561 ) ) ;
#31909=CARTESIAN_POINT ( 'NONE',  ( -1.909035429704832693E-15, 195.8375000000000057, -31.17691453623979214 ) ) ;
#32010=CARTESIAN_POINT ( 'NONE',  ( -27.00000000000000355, 196.5125000012290570, 0.000000000000000000 ) ) ;
#32028=CARTESIAN_POINT ( 'NONE',  ( 5.778771075727756162E-15, 196.8218750006145399, 31.45816453501075927 ) ) ;
#32053=CARTESIAN_POINT ( 'NONE',  ( 13.62178482187499640, 198.7531250006145456, -23.59362340125807123 ) ) ;
#32072=ORIENTED_EDGE ( 'NONE', *, *, #19573, .F. ) ;
#32077=CARTESIAN_POINT ( 'NONE',  ( -13.62178482187500528, 196.1843750006145228, -23.59362340125807123 ) ) ;
#32081=( BOUNDED_CURVE ( )  B_SPLINE_CURVE ( 2, ( #8964, #26577, #23560, #31892, #22817, #2704, #17690, #34365, #28856 ),
 .UNSPECIFIED., .F., .F. ) 
 B_SPLINE_CURVE_WITH_KNOTS ( ( 3, 2, 2, 2, 3 ),
 ( 0.2291666666666666574, 0.2361111111111111049, 0.2500000000000000000, 0.2638888888888888951, 0.2708333333333333703 ),
 .UNSPECIFIED. ) 
 CURVE ( )  GEOMETRIC_REPRESENTATION_ITEM ( )  RATIONAL_B_SPLINE_CURVE ( ( 0.9330127018922194093, 0.9330127018922194093, 1.000000000000000000, 0.8660254037844387076, 1.000000000000000000, 0.8660254037844387076, 1.000000000000000000, 0.9330127018922190762, 0.9330127018922194093 ) ) 
 REPRESENTATION_ITEM ( '' )  );
#32085=VERTEX_POINT ( 'NONE', #20210 ) ;
#32089=EDGE_CURVE ( 'NONE', #26752, #32409, #90, .T. ) ;
#32093=CARTESIAN_POINT ( 'NONE',  ( -13.62178482187500528, 198.8843750006145399, -23.59362340125807123 ) ) ;
#32096=ORIENTED_EDGE ( 'NONE', *, *, #20765, .F. ) ;
#32120=CARTESIAN_POINT ( 'NONE',  ( -7.234628195640354420, 194.8049038117966916, 26.99999999999996803 ) ) ;
#32125=FACE_OUTER_BOUND ( 'NONE', #33270, .T. ) ;
#32162=VERTEX_POINT ( 'NONE', #18117 ) ;
#32174=LINE ( 'NONE', #31615, #7994 ) ;
#32178=CARTESIAN_POINT ( 'NONE',  ( 13.50000000000001421, 199.7000000000000171, 23.38268590217984055 ) ) ;
#32202=CARTESIAN_POINT ( 'NONE',  ( -1.909035429704832693E-15, 195.5000000012290400, -31.17691453623979214 ) ) ;
#32220=CARTESIAN_POINT ( 'NONE',  ( 27.24356964375000345, 195.5843750006145285, -3.336375036156643733E-15 ) ) ;
#32241=CARTESIAN_POINT ( 'NONE',  ( 27.24356964375000700, 198.6406250006145058, 15.72908226750537075 ) ) ;
#32262=CARTESIAN_POINT ( 'NONE',  ( 27.24356964375000345, 195.1343750006145399, -3.336375036156643733E-15 ) ) ;
#32278=CARTESIAN_POINT ( 'NONE',  ( -13.62178482187500528, 198.4343750006145228, -23.59362340125807123 ) ) ;
#32326=CARTESIAN_POINT ( 'NONE',  ( 26.99999999999999645, 199.8125000000000000, -15.58845726811990495 ) ) ;
#32329=VERTEX_POINT ( 'NONE', #32498 ) ;
#32340=DIRECTION ( 'NONE',  ( -0.000000000000000000, -1.000000000000000000, -0.000000000000000000 ) ) ;
#32361=DIRECTION ( 'NONE',  ( -0.000000000000000000, -1.000000000000000000, -0.000000000000000000 ) ) ;
#32376=ADVANCED_FACE ( 'NONE', ( #26826 ), #10330, .T. ) ;
#32386=CARTESIAN_POINT ( 'NONE',  ( 27.00000000000000355, 197.1875000012290400, -3.306546357697854128E-15 ) ) ;
#32407=CARTESIAN_POINT ( 'NONE',  ( -1.926257025242585782E-15, 195.6968750006145683, -31.45816453501075927 ) ) ;
#32409=VERTEX_POINT ( 'NONE', #29856 ) ;
#32418=CARTESIAN_POINT ( 'NONE',  ( 27.24356964375000345, 198.7343750006145626, -3.336375036156643733E-15 ) ) ;
#32419=ORIENTED_EDGE ( 'NONE', *, *, #23148, .F. ) ;
#32429=CARTESIAN_POINT ( 'NONE',  ( -27.24356964374999635, 199.3906250006145342, 15.72908226750539384 ) ) ;
#32450=CARTESIAN_POINT ( 'NONE',  ( 1.120210788295102201E-13, 195.3875000000000455, -27.00000000000000711 ) ) ;
#32452=CARTESIAN_POINT ( 'NONE',  ( -13.62178482187498396, 199.4281250006145569, 23.59362340125808188 ) ) ;
#32453=DIRECTION ( 'NONE',  ( 0.000000000000000000, 0.000000000000000000, -1.000000000000000000 ) ) ;
#32467=CARTESIAN_POINT ( 'NONE',  ( 27.24356964375000700, 197.7968750006145342, 15.72908226750537075 ) ) ;
#32498=CARTESIAN_POINT ( 'NONE',  ( -3.253724281355068545E-15, 197.6374999999999602, -27.00000000000000355 ) ) ;
#32504=CARTESIAN_POINT ( 'NONE',  ( 13.50000000000001421, 197.4500000000000171, 23.38268590217984055 ) ) ;
#32509=DIRECTION ( 'NONE',  ( -0.000000000000000000, -1.000000000000000000, -0.000000000000000000 ) ) ;
#32564=VERTEX_POINT ( 'NONE', #15464 ) ;
#32595=CARTESIAN_POINT ( 'NONE',  ( 13.62178482187499640, 195.2093750006145569, -23.59362340125807123 ) ) ;
#32604=CARTESIAN_POINT ( 'NONE',  ( 27.00000000000001421, 199.4000000012290457, 15.58845726811988897 ) ) ;
#32607=CARTESIAN_POINT ( 'NONE',  ( 27.24356964375000700, 198.2468750006145513, 15.72908226750537075 ) ) ;
#32621=CARTESIAN_POINT ( 'NONE',  ( -27.24356964374999990, 197.5156250006145626, -15.72908226750537786 ) ) ;
#32630=ORIENTED_EDGE ( 'NONE', *, *, #19158, .T. ) ;
#32643=CARTESIAN_POINT ( 'NONE',  ( -27.24356964375000345, 197.5531250006145285, 0.000000000000000000 ) ) ;
#32645=CARTESIAN_POINT ( 'NONE',  ( 3.306546357697854128E-15, 200.0000000000000000, 27.00000000000000355 ) ) ;
#32658=CARTESIAN_POINT ( 'NONE',  ( 5.778771075727756162E-15, 197.2718750006145569, 31.45816453501075927 ) ) ;
#32659=ORIENTED_EDGE ( 'NONE', *, *, #15166, .F. ) ;
#32667=FACE_OUTER_BOUND ( 'NONE', #16274, .T. ) ;
#32682=CARTESIAN_POINT ( 'NONE',  ( 13.62178482187499640, 197.8531250006145399, -23.59362340125807123 ) ) ;
#32692=VERTEX_POINT ( 'NONE', #4636 ) ;
#32699=CARTESIAN_POINT ( 'NONE',  ( 0.000000000000000000, 200.0000000000000000, -27.00000000000000355 ) ) ;
#32700=EDGE_CURVE ( 'NONE', #26583, #29410, #20821, .T. ) ;
#32785=CARTESIAN_POINT ( 'NONE',  ( 5.778771075727756162E-15, 195.4718750006145456, 31.45816453501075927 ) ) ;
#32796=CARTESIAN_POINT ( 'NONE',  ( -27.24356964375000345, 198.0218750006145569, -15.72908226750537786 ) ) ;
#32805=VERTEX_POINT ( 'NONE', #10709 ) ;
#32807=CARTESIAN_POINT ( 'NONE',  ( 13.62178482187499640, 195.6031250006145115, -23.59362340125807123 ) ) ;
#32830=CARTESIAN_POINT ( 'NONE',  ( 27.24356964375000345, 198.2281250006145399, -3.336375036156643733E-15 ) ) ;
#32873=CARTESIAN_POINT ( 'NONE',  ( 27.24356964374999279, 197.3656250006145285, -15.72908226750539207 ) ) ;
#32889=CARTESIAN_POINT ( 'NONE',  ( -27.00000000000000355, 199.0625000000000000, -15.58845726811989429 ) ) ;
#32896=DIRECTION ( 'NONE',  ( -0.000000000000000000, -1.000000000000000000, -0.000000000000000000 ) ) ;
#32926=AXIS2_PLACEMENT_3D ( 'NONE', #18508, #10144, #33448 ) ;
#32941=ORIENTED_EDGE ( 'NONE', *, *, #33716, .F. ) ;
#32984=CARTESIAN_POINT ( 'NONE',  ( -1.926257025242585782E-15, 196.1468750006145569, -31.45816453501076637 ) ) ;
#32997=CARTESIAN_POINT ( 'NONE',  ( -27.24356964375000345, 197.5531250006145285, 0.000000000000000000 ) ) ;
#33023=CARTESIAN_POINT ( 'NONE',  ( -27.24356964374999635, 198.9406250006145171, 15.72908226750539384 ) ) ;
#33049=CARTESIAN_POINT ( 'NONE',  ( 0.000000000000000000, 200.0000000000000000, 0.000000000000000000 ) ) ;
#33066=CARTESIAN_POINT ( 'NONE',  ( -13.62178482187498396, 197.1781250006145569, 23.59362340125808188 ) ) ;
#33068=( BOUNDED_CURVE ( )  B_SPLINE_CURVE ( 2, ( #36918, #27659, #1684, #10410, #5089, #28214, #13259, #4715, #36550 ),
 .UNSPECIFIED., .F., .F. ) 
 B_SPLINE_CURVE_WITH_KNOTS ( ( 3, 2, 2, 2, 3 ),
 ( 0.7291666666666667407, 0.7361111111111111605, 0.7500000000000000000, 0.7638888888888888395, 0.7708333333333333703 ),
 .UNSPECIFIED. ) 
 CURVE ( )  GEOMETRIC_REPRESENTATION_ITEM ( )  RATIONAL_B_SPLINE_CURVE ( ( 0.9330127018922192983, 0.9330127018922198534, 1.000000000000000000, 0.8660254037844387076, 1.000000000000000000, 0.8660254037844387076, 1.000000000000000000, 0.9330127018922187432, 0.9330127018922192983 ) ) 
 REPRESENTATION_ITEM ( '' )  );
#33083=CARTESIAN_POINT ( 'NONE',  ( -26.99999999999998934, 198.2374999999999829, 15.58845726811991561 ) ) ;
#33138=ORIENTED_EDGE ( 'NONE', *, *, #27314, .T. ) ;
#33155=CARTESIAN_POINT ( 'NONE',  ( -1.045839947578415010E-13, 196.0625000000000284, 27.00000000000000355 ) ) ;
#33168=CIRCLE ( 'NONE', #34962, 25.00000000000000000 ) ;
#33177=CARTESIAN_POINT ( 'NONE',  ( -27.24356964375000345, 196.7093750006145569, 0.000000000000000000 ) ) ;
#33178=ORIENTED_EDGE ( 'NONE', *, *, #19803, .T. ) ;
#33179=ORIENTED_EDGE ( 'NONE', *, *, #1371, .T. ) ;
#33186=VERTEX_POINT ( 'NONE', #37460 ) ;
#33189=CARTESIAN_POINT ( 'NONE',  ( -1.926257025242585782E-15, 196.0906250006145228, -31.45816453501075927 ) ) ;
#33199=EDGE_CURVE ( 'NONE', #10880, #2775, #22719, .T. ) ;
#33202=CARTESIAN_POINT ( 'NONE',  ( 1.120210788295102201E-13, 195.5000000012290400, -27.00000000000000711 ) ) ;
#33214=CARTESIAN_POINT ( 'NONE',  ( -27.24356964374999635, 198.0406250006145399, 15.72908226750539384 ) ) ;
#33248=CARTESIAN_POINT ( 'NONE',  ( -27.00000000000000355, 197.3750000012290400, -15.58845726811989429 ) ) ;
#33251=CARTESIAN_POINT ( 'NONE',  ( 13.62178482187499640, 198.7531250006145456, -23.59362340125807123 ) ) ;
#33269=CARTESIAN_POINT ( 'NONE',  ( -27.00000000000000355, 197.3000000000000114, 0.000000000000000000 ) ) ;
#33270=EDGE_LOOP ( 'NONE', ( #3264, #15659, #4371, #31678 ) ) ;
#33324=ORIENTED_EDGE ( 'NONE', *, *, #15199, .T. ) ;
#33332=CARTESIAN_POINT ( 'NONE',  ( 13.50000000000001421, 195.3125000012290400, 23.38268590217984055 ) ) ;
#33364=CARTESIAN_POINT ( 'NONE',  ( -27.24356964375000345, 197.1218750006145513, -15.72908226750537786 ) ) ;
#33376=CARTESIAN_POINT ( 'NONE',  ( -13.62178482187498396, 196.2781250006145228, 23.59362340125808188 ) ) ;
#33384=LINE ( 'NONE', #19552, #10351 ) ;
#33389=CARTESIAN_POINT ( 'NONE',  ( 13.50000000000001421, 195.3125000012290400, 23.38268590217984055 ) ) ;
#33392=CARTESIAN_POINT ( 'NONE',  ( 13.50000000000001421, 199.2500000000000000, 23.38268590217984055 ) ) ;
#33394=B_SPLINE_CURVE_WITH_KNOTS ( 'NONE', 3,
 ( #35251, #18406, #6644, #9305 ),
 .UNSPECIFIED., .F., .F.,
 ( 4, 4 ),
 ( 0.000000000000000000, 1.000000000000000000 ),
 .UNSPECIFIED. ) ;
#33400=CARTESIAN_POINT ( 'NONE',  ( -1.926257025242585782E-15, 195.1906250006145456, -31.45816453501075927 ) ) ;
#33406=ORIENTED_EDGE ( 'NONE', *, *, #19711, .T. ) ;
#33414=ORIENTED_EDGE ( 'NONE', *, *, #29259, .T. ) ;
#33434=CARTESIAN_POINT ( 'NONE',  ( 13.62178482187499640, 197.4031250006145228, -23.59362340125807123 ) ) ;
#33439=CARTESIAN_POINT ( 'NONE',  ( -1.045839947578415010E-13, 196.1750000012290229, 27.00000000000000355 ) ) ;
#33448=DIRECTION ( 'NONE',  ( 0.000000000000000000, 0.000000000000000000, -1.000000000000000000 ) ) ;
#33449=CARTESIAN_POINT ( 'NONE',  ( -13.50000000000000533, 197.6750000000000114, -23.38268590217984411 ) ) ;
#33515=CARTESIAN_POINT ( 'NONE',  ( -27.00000000000000355, 199.5500000000000114, 0.000000000000000000 ) ) ;
#33555=( GEOMETRIC_REPRESENTATION_CONTEXT ( 3 ) GLOBAL_UNCERTAINTY_ASSIGNED_CONTEXT ( ( #4786 ) ) GLOBAL_UNIT_ASSIGNED_CONTEXT ( ( #19083, #36298, #25491 ) ) REPRESENTATION_CONTEXT ( 'NONE', 'WORKASPACE' ) );
#33564=CARTESIAN_POINT ( 'NONE',  ( 27.00000000000001066, 199.4000000012290172, 15.58845726811988897 ) ) ;
#33586=CARTESIAN_POINT ( 'NONE',  ( -27.24356964375000345, 195.7531250006145456, 0.000000000000000000 ) ) ;
#33589=EDGE_CURVE ( 'NONE', #22836, #24000, #32081, .T. ) ;
#33625=CARTESIAN_POINT ( 'NONE',  ( -1.926257025242585782E-15, 195.1906250006145456, -31.45816453501076637 ) ) ;
#33626=CARTESIAN_POINT ( 'NONE',  ( -27.24356964375000345, 198.9593750006145285, 0.000000000000000000 ) ) ;
#33629=CARTESIAN_POINT ( 'NONE',  ( -1.045839947578415010E-13, 195.1625000000000512, 27.00000000000000355 ) ) ;
#33641=CARTESIAN_POINT ( 'NONE',  ( -27.00000000000000355, 198.2000000000000171, 0.000000000000000000 ) ) ;
#33645=EDGE_LOOP ( 'NONE', ( #26499, #3097, #13182, #15898, #17667, #20111, #33324, #34296, #5175, #33179, #31815, #31379, #36245, #23193, #4571, #23810, #4454, #5839, #14893, #19536, #13303, #35961, #33406, #29484, #37073, #30793 ) ) ;
#33648=DIRECTION ( 'NONE',  ( -0.000000000000000000, -1.000000000000000000, -0.000000000000000000 ) ) ;
#33689=DIRECTION ( 'NONE',  ( -0.000000000000000000, -1.000000000000000000, -0.000000000000000000 ) ) ;
#33694=ORIENTED_EDGE ( 'NONE', *, *, #2642, .T. ) ;
#33716=EDGE_CURVE ( 'NONE', #4030, #22836, #24503, .T. ) ;
#33735=CARTESIAN_POINT ( 'NONE',  ( -1.926257025242585782E-15, 195.6968750006145683, -31.45816453501076637 ) ) ;
#33748=CARTESIAN_POINT ( 'NONE',  ( -27.24356964374999635, 194.8906250006145342, 15.72908226750539384 ) ) ;
#33773=CARTESIAN_POINT ( 'NONE',  ( -27.24356964374999990, 195.7156250006145513, -15.72908226750537786 ) ) ;
#33788=ORIENTED_EDGE ( 'NONE', *, *, #31566, .F. ) ;
#33813=CARTESIAN_POINT ( 'NONE',  ( -13.62178482187498396, 195.8281250006145342, 23.59362340125808188 ) ) ;
#33814=CARTESIAN_POINT ( 'NONE',  ( -27.24356964374999635, 198.9968750006145228, 15.72908226750539384 ) ) ;
#33817=DIRECTION ( 'NONE',  ( -0.000000000000000000, -1.000000000000000000, -0.000000000000000000 ) ) ;
#33830=CARTESIAN_POINT ( 'NONE',  ( 13.50000000000001421, 197.4500000000000171, 23.38268590217984055 ) ) ;
#33834=EDGE_LOOP ( 'NONE', ( #37439, #12041, #30897, #17608 ) ) ;
#33881=ORIENTED_EDGE ( 'NONE', *, *, #13054, .T. ) ;
#33882=ORIENTED_EDGE ( 'NONE', *, *, #31144, .T. ) ;
#33889=CARTESIAN_POINT ( 'NONE',  ( -7.234628195640302017, 199.6424038105676857, 27.00000000000000711 ) ) ;
#33901=CARTESIAN_POINT ( 'NONE',  ( -13.50000000000000533, 197.6750000000000114, -23.38268590217984411 ) ) ;
#33909=ORIENTED_EDGE ( 'NONE', *, *, #26807, .T. ) ;
#33931=CARTESIAN_POINT ( 'NONE',  ( -1.926257025242585782E-15, 195.1906250006145456, -31.45816453501075927 ) ) ;
#33953=CARTESIAN_POINT ( 'NONE',  ( -1.926257025242585782E-15, 196.5406250006145399, -31.45816453501075927 ) ) ;
#33961=VERTEX_POINT ( 'NONE', #13692 ) ;
#33971=CARTESIAN_POINT ( 'NONE',  ( -7.234628195640313564, 199.9075961894323541, -27.00000000000000355 ) ) ;
#33980=DIRECTION ( 'NONE',  ( -0.000000000000000000, -1.000000000000000000, -0.000000000000000000 ) ) ;
#33988=CARTESIAN_POINT ( 'NONE',  ( 1.120210788295102201E-13, 195.0500000012290798, -27.00000000000000711 ) ) ;
#33991=CARTESIAN_POINT ( 'NONE',  ( -27.24356964374999279, 196.2406250006145285, 15.72908226750539384 ) ) ;
#33992=CARTESIAN_POINT ( 'NONE',  ( 13.62178482187499640, 198.3593750006145342, -23.59362340125807123 ) ) ;
#33995=CARTESIAN_POINT ( 'NONE',  ( 0.000000000000000000, 2.000000000000000000, 0.000000000000000000 ) ) ;
#34008=CARTESIAN_POINT ( 'NONE',  ( 26.99999999999999645, 195.3125000000000284, -15.58845726811990495 ) ) ;
#34024=( LENGTH_UNIT ( ) NAMED_UNIT ( * ) SI_UNIT ( .MILLI., .METRE. ) );
#34035=ORIENTED_EDGE ( 'NONE', *, *, #26389, .T. ) ;
#34089=CARTESIAN_POINT ( 'NONE',  ( 0.000000000000000000, 200.0000000000000000, 0.000000000000000000 ) ) ;
#34113=CARTESIAN_POINT ( 'NONE',  ( -27.00000000000000355, 199.2125000012290457, 0.000000000000000000 ) ) ;
#34134=CYLINDRICAL_SURFACE ( 'NONE', #19775, 27.00000000000000355 ) ;
#34135=STYLED_ITEM('',(#37556),#7452);
#34139=CARTESIAN_POINT ( 'NONE',  ( 13.62178482187501416, 197.2531250006145456, 23.59362340125806767 ) ) ;
#34142=CARTESIAN_POINT ( 'NONE',  ( 0.000000000000000000, 200.0000000000000000, 0.000000000000000000 ) ) ;
#34146=ORIENTED_EDGE ( 'NONE', *, *, #31242, .F. ) ;
#34167=CARTESIAN_POINT ( 'NONE',  ( -26.99999999999999645, 196.8875000000000171, 15.58845726811991561 ) ) ;
#34179=CARTESIAN_POINT ( 'NONE',  ( 5.778771075727756162E-15, 196.3156250006145171, 31.45816453501076637 ) ) ;
#34180=ADVANCED_FACE ( 'NONE', ( #27714 ), #11022, .T. ) ;
#34181=CARTESIAN_POINT ( 'NONE',  ( 13.62178482187499640, 197.9093750006145456, -23.59362340125807123 ) ) ;
#34183=CARTESIAN_POINT ( 'NONE',  ( 27.00000000000001421, 195.6875000000000000, 15.58845726811988897 ) ) ;
#34184=CARTESIAN_POINT ( 'NONE',  ( 13.50000000000001421, 196.2125000012290172, 23.38268590217984055 ) ) ;
#34196=CARTESIAN_POINT ( 'NONE',  ( 27.00000000000000355, 195.2750000000000057, -3.306546357697854128E-15 ) ) ;
#34251=ORIENTED_EDGE ( 'NONE', *, *, #21488, .T. ) ;
#34288=( BOUNDED_CURVE ( )  B_SPLINE_CURVE ( 2, ( #6591, #21202, #29706, #333, #26673, #6403, #32178, #6214, #11711 ),
 .UNSPECIFIED., .F., .F. ) 
 B_SPLINE_CURVE_WITH_KNOTS ( ( 3, 2, 2, 2, 3 ),
 ( 0.02083333333333333565, 0.02777777777777777624, 0.04166666666666666435, 0.05555555555555555247, 0.06250000000000000000 ),
 .UNSPECIFIED. ) 
 CURVE ( )  GEOMETRIC_REPRESENTATION_ITEM ( )  RATIONAL_B_SPLINE_CURVE ( ( 0.9330127018922194093, 0.9330127018922194093, 1.000000000000000000, 0.8660254037844387076, 1.000000000000000000, 0.8660254037844387076, 1.000000000000000000, 0.9330127018922194093, 0.9330127018922194093 ) ) 
 REPRESENTATION_ITEM ( '' )  );
#34294=CARTESIAN_POINT ( 'NONE',  ( 13.62178482187501416, 195.5093750006145399, 23.59362340125806767 ) ) ;
#34296=ORIENTED_EDGE ( 'NONE', *, *, #33589, .T. ) ;
#34302=CARTESIAN_POINT ( 'NONE',  ( 26.99999999999999645, 199.4750000012290343, -15.58845726811990495 ) ) ;
#34324=CARTESIAN_POINT ( 'NONE',  ( -20.86978604919638869, 194.8026013911397740, -17.51182792271053046 ) ) ;
#34329=EDGE_CURVE ( 'NONE', #22009, #13180, #13807, .T. ) ;
#34351=CARTESIAN_POINT ( 'NONE',  ( -20.68320042480036491, 194.9994763866750134, -17.35526491262920246 ) ) ;
#34353=CYLINDRICAL_SURFACE ( 'NONE', #5230, 27.00000000000000355 ) ;
#34363=CARTESIAN_POINT ( 'NONE',  ( 13.62178482187501416, 197.3093750006145513, 23.59362340125806767 ) ) ;
#34365=CARTESIAN_POINT ( 'NONE',  ( -7.234628195640289583, 198.5575961894323029, -27.00000000000001421 ) ) ;
#34366=CARTESIAN_POINT ( 'NONE',  ( 0.000000000000000000, 200.0000000000000000, 0.000000000000000000 ) ) ;
#34382=CARTESIAN_POINT ( 'NONE',  ( -27.24356964374999990, 199.3718750006145513, -15.72908226750537786 ) ) ;
#34385=EDGE_LOOP ( 'NONE', ( #1139, #9214, #25838, #16299 ) ) ;
#34418=DIRECTION ( 'NONE',  ( 0.000000000000000000, 1.000000000000000000, 0.000000000000000000 ) ) ;
#34437=DIRECTION ( 'NONE',  ( 0.000000000000000000, 0.000000000000000000, -1.000000000000000000 ) ) ;
#34459=CARTESIAN_POINT ( 'NONE',  ( -7.234628195640328663, 197.0549038117967484, 26.99999999999999289 ) ) ;
#34463=CARTESIAN_POINT ( 'NONE',  ( -13.50000000000000533, 197.2250000000000227, -23.38268590217984411 ) ) ;
#34485=CARTESIAN_POINT ( 'NONE',  ( -13.50000000000000533, 196.4375000012290400, -23.38268590217984411 ) ) ;
#34489=EDGE_CURVE ( 'NONE', #3136, #9546, #5727, .T. ) ;
#34504=VECTOR ( 'NONE', #13072, 1000.000000000000000 ) ;
#34537=FACE_OUTER_BOUND ( 'NONE', #27953, .T. ) ;
#34546=CARTESIAN_POINT ( 'NONE',  ( -13.62178482187500528, 195.7343750006145626, -23.59362340125807123 ) ) ;
#34547=DIRECTION ( 'NONE',  ( 0.000000000000000000, -1.000000000000000000, 0.000000000000000000 ) ) ;
#34557=CARTESIAN_POINT ( 'NONE',  ( -7.234628195640263826, 195.8575961894323711, -27.00000000000003553 ) ) ;
#34565=CARTESIAN_POINT ( 'NONE',  ( 27.24356964374999635, 199.2218750006145456, -15.72908226750539029 ) ) ;
#34600=CARTESIAN_POINT ( 'NONE',  ( 5.438367727407757144E-14, 197.7500000012290400, -27.00000000000000000 ) ) ;
#34666=CARTESIAN_POINT ( 'NONE',  ( -27.00000000000000355, 197.3750000012290400, -15.58845726811989429 ) ) ;
#34685=VERTEX_POINT ( 'NONE', #12522 ) ;
#34706=CARTESIAN_POINT ( 'NONE',  ( -13.62178482187498396, 199.4281250006145569, 23.59362340125808188 ) ) ;
#34728=EDGE_LOOP ( 'NONE', ( #3510, #35865 ) ) ;
#34731=CARTESIAN_POINT ( 'NONE',  ( -27.24356964374999990, 196.2218750006145456, -15.72908226750537786 ) ) ;
#34743=CARTESIAN_POINT ( 'NONE',  ( 13.49999999999999645, 197.2625000012290286, -23.38268590217984766 ) ) ;
#34745=EDGE_LOOP ( 'NONE', ( #35624, #6127, #35098, #29021 ) ) ;
#34751=CARTESIAN_POINT ( 'NONE',  ( -13.49999999999998401, 195.1250000000000284, 23.38268590217985476 ) ) ;
#34779=CARTESIAN_POINT ( 'NONE',  ( -27.24356964374999279, 198.9406250006145171, 15.72908226750539384 ) ) ;
#34798=VERTEX_POINT ( 'NONE', #16681 ) ;
#34831=CARTESIAN_POINT ( 'NONE',  ( 1.069080835302379631E-14, 198.4250000012290229, 27.00000000000000000 ) ) ;
#34853=CARTESIAN_POINT ( 'NONE',  ( 5.727106289114498080E-15, 196.6250000012290400, 31.17691453623979214 ) ) ;
#34859=EDGE_CURVE ( 'NONE', #10453, #17469, #33168, .T. ) ;
#34870=CARTESIAN_POINT ( 'NONE',  ( 13.50000000000001421, 196.6625000012290343, 23.38268590217984055 ) ) ;
#34873=CARTESIAN_POINT ( 'NONE',  ( 13.62178482187501416, 195.9593750006145569, 23.59362340125806767 ) ) ;
#34880=EDGE_CURVE ( 'NONE', #21721, #36421, #25383, .T. ) ;
#34918=CARTESIAN_POINT ( 'NONE',  ( -27.24356964374999990, 197.1218750006145228, -15.72908226750537786 ) ) ;
#34926=ORIENTED_EDGE ( 'NONE', *, *, #9709, .F. ) ;
#34934=CARTESIAN_POINT ( 'NONE',  ( 27.24356964375000345, 196.9343750006145228, -3.336375036156643733E-15 ) ) ;
#34962=AXIS2_PLACEMENT_3D ( 'NONE', #2257, #13647, #36375 ) ;
#34964=CARTESIAN_POINT ( 'NONE',  ( -13.49999999999998401, 194.7875000012290343, 23.38268590217985476 ) ) ;
#34982=CARTESIAN_POINT ( 'NONE',  ( 13.50000000000001421, 199.7000000000000171, 23.38268590217984055 ) ) ;
#34985=AXIS2_PLACEMENT_3D ( 'NONE', #20678, #25606, #17842 ) ;
#34990=PRODUCT_DEFINITION_CONTEXT ( 'detailed design', #11249, 'design' ) ;
#35039=CARTESIAN_POINT ( 'NONE',  ( 27.00000000000000355, 195.8375000012290457, -3.306546357697854128E-15 ) ) ;
#35057=CARTESIAN_POINT ( 'NONE',  ( -13.62178482187498396, 195.4343750006145228, 23.59362340125808188 ) ) ;
#35080=CARTESIAN_POINT ( 'NONE',  ( 13.62178482187501416, 198.1531250006145228, 23.59362340125806767 ) ) ;
#35098=ORIENTED_EDGE ( 'NONE', *, *, #18426, .F. ) ;
#35103=CARTESIAN_POINT ( 'NONE',  ( -13.62178482187498396, 195.4343750006145228, 23.59362340125808188 ) ) ;
#35104=CARTESIAN_POINT ( 'NONE',  ( 0.000000000000000000, 200.0000000000000000, 0.000000000000000000 ) ) ;
#35110=LINE ( 'NONE', #20725, #20894 ) ;
#35119=CARTESIAN_POINT ( 'NONE',  ( -27.24356964375000345, 198.5093750006145399, 0.000000000000000000 ) ) ;
#35170=CARTESIAN_POINT ( 'NONE',  ( -7.234628195640289583, 198.2200961906613372, -27.00000000000001421 ) ) ;
#35209=CARTESIAN_POINT ( 'NONE',  ( 7.234628195640269155, 196.5325961894323257, 27.00000000000003197 ) ) ;
#35225=CARTESIAN_POINT ( 'NONE',  ( 5.727106289114498080E-15, 195.7250000012290343, 31.17691453623979214 ) ) ;
#35243=CARTESIAN_POINT ( 'NONE',  ( 27.24356964374999635, 195.6218750006145228, -15.72908226750539029 ) ) ;
#35250=FACE_OUTER_BOUND ( 'NONE', #2005, .T. ) ;
#35251=CARTESIAN_POINT ( 'NONE',  ( -20.68320086892770604, 194.6619763917542798, -17.35526438333879540 ) ) ;
#35253=CARTESIAN_POINT ( 'NONE',  ( -1.926257025242585782E-15, 198.8468750006145740, -31.45816453501076637 ) ) ;
#35263=CARTESIAN_POINT ( 'NONE',  ( 27.24356964374999635, 197.8156250006145171, -15.72908226750539029 ) ) ;
#35269=CARTESIAN_POINT ( 'NONE',  ( 1.120210788295102201E-13, 197.1875000000000568, -27.00000000000000711 ) ) ;
#35285=CARTESIAN_POINT ( 'NONE',  ( 13.62178482187501416, 198.1531250006145228, 23.59362340125806767 ) ) ;
#35286=CARTESIAN_POINT ( 'NONE',  ( 7.234628195640322446, 197.9950961906613429, 26.99999999999999645 ) ) ;
#35301=CARTESIAN_POINT ( 'NONE',  ( -13.62178482187500528, 197.9843750006145626, -23.59362340125807123 ) ) ;
#35323=CARTESIAN_POINT ( 'NONE',  ( -3.253724281355068545E-15, 198.9874999999999829, -27.00000000000000355 ) ) ;
#35343=CARTESIAN_POINT ( 'NONE',  ( 26.99999999999999645, 197.5625000000000000, -15.58845726811990495 ) ) ;
#35356=DIRECTION ( 'NONE',  ( 0.000000000000000000, 0.000000000000000000, -1.000000000000000000 ) ) ;
#35363=DIRECTION ( 'NONE',  ( 0.000000000000000000, 1.000000000000000000, 0.000000000000000000 ) ) ;
#35429=CARTESIAN_POINT ( 'NONE',  ( -3.253724281355068545E-15, 198.9874999999999829, -27.00000000000000000 ) ) ;
#35433=CARTESIAN_POINT ( 'NONE',  ( -13.62178482187498396, 196.3343750006145285, 23.59362340125808188 ) ) ;
#35443=CARTESIAN_POINT ( 'NONE',  ( 1.069080835302379631E-14, 198.3124999999999716, 27.00000000000000000 ) ) ;
#35445=CARTESIAN_POINT ( 'NONE',  ( -13.62178482187500528, 197.9843750006145626, -23.59362340125807123 ) ) ;
#35456=ORIENTED_EDGE ( 'NONE', *, *, #20976, .F. ) ;
#35457=CARTESIAN_POINT ( 'NONE',  ( 27.24356964374999635, 195.5656250006145171, -15.72908226750539029 ) ) ;
#35464=CARTESIAN_POINT ( 'NONE',  ( 1.069080835302379631E-14, 196.9624999999999773, 27.00000000000000000 ) ) ;
#35475=EDGE_CURVE ( 'NONE', #37126, #5600, #14936, .T. ) ;
#35481=CARTESIAN_POINT ( 'NONE',  ( 5.778771075727756162E-15, 199.0156250006145342, 31.45816453501075927 ) ) ;
#35495=CARTESIAN_POINT ( 'NONE',  ( 13.62178482187499640, 197.0093750006145399, -23.59362340125807123 ) ) ;
#35497=EDGE_LOOP ( 'NONE', ( #14287, #34035, #204, #19596 ) ) ;
#35518=FACE_OUTER_BOUND ( 'NONE', #18338, .T. ) ;
#35526=CARTESIAN_POINT ( 'NONE',  ( -27.24356964375000345, 196.6156250006145285, -15.72908226750537786 ) ) ;
#35563=LINE ( 'NONE', #13017, #6426 ) ;
#35581=CYLINDRICAL_SURFACE ( 'NONE', #3863, 27.00000000000000355 ) ;
#35606=AXIS2_PLACEMENT_3D ( 'NONE', #1023, #4431, #9380 ) ;
#35622=CARTESIAN_POINT ( 'NONE',  ( -1.926257025242585782E-15, 196.5968750006145456, -31.45816453501075927 ) ) ;
#35624=ORIENTED_EDGE ( 'NONE', *, *, #5546, .T. ) ;
#35631=CARTESIAN_POINT ( 'NONE',  ( 1.069080835302379631E-14, 198.7624999999999886, 27.00000000000000000 ) ) ;
#35633=CARTESIAN_POINT ( 'NONE',  ( 5.778771075727756162E-15, 196.3718750006145513, 31.45816453501076637 ) ) ;
#35647=CARTESIAN_POINT ( 'NONE',  ( 5.778771075727756162E-15, 196.3156250006145171, 31.45816453501075927 ) ) ;
#35670=CARTESIAN_POINT ( 'NONE',  ( 5.778771075727756162E-15, 199.4656250006145797, 31.45816453501075927 ) ) ;
#35708=CARTESIAN_POINT ( 'NONE',  ( -13.62178482187498396, 198.0781250006145342, 23.59362340125808188 ) ) ;
#35718=VECTOR ( 'NONE', #16342, 1000.000000000000000 ) ;
#35728=ORIENTED_EDGE ( 'NONE', *, *, #21488, .F. ) ;
#35733=CYLINDRICAL_SURFACE ( 'NONE', #21982, 27.00000000000000355 ) ;
#35820=FACE_OUTER_BOUND ( 'NONE', #4349, .T. ) ;
#35822=CARTESIAN_POINT ( 'NONE',  ( -27.24356964374999279, 196.2968750006145342, 15.72908226750539384 ) ) ;
#35823=ORIENTED_EDGE ( 'NONE', *, *, #23982, .F. ) ;
#35835=CARTESIAN_POINT ( 'NONE',  ( -13.62178482187498396, 196.7281250006145399, 23.59362340125808188 ) ) ;
#35858=CARTESIAN_POINT ( 'NONE',  ( 27.24356964375000345, 199.5781250006145342, -3.336375036156643733E-15 ) ) ;
#35865=ORIENTED_EDGE ( 'NONE', *, *, #34859, .F. ) ;
#35889=CARTESIAN_POINT ( 'NONE',  ( -13.50000000000000533, 198.1250000000000284, -23.38268590217984411 ) ) ;
#35897=CARTESIAN_POINT ( 'NONE',  ( 27.24356964375000700, 197.7406250006145285, 15.72908226750537075 ) ) ;
#35898=CARTESIAN_POINT ( 'NONE',  ( -27.24356964375000345, 199.8593750006145342, 0.000000000000000000 ) ) ;
#35913=CARTESIAN_POINT ( 'NONE',  ( -27.00000000000000355, 197.7500000000000000, 0.000000000000000000 ) ) ;
#35961=ORIENTED_EDGE ( 'NONE', *, *, #25994, .T. ) ;
#35980=AXIS2_PLACEMENT_3D ( 'NONE', #33995, #13537, #36832 ) ;
#36011=CARTESIAN_POINT ( 'NONE',  ( -27.24356964375000345, 198.0593750006145513, 0.000000000000000000 ) ) ;
#36022=CARTESIAN_POINT ( 'NONE',  ( 13.62178482187501416, 195.4531250006145342, 23.59362340125806767 ) ) ;
#36028=ADVANCED_FACE ( 'NONE', ( #20418 ), #11501, .T. ) ;
#36034=CARTESIAN_POINT ( 'NONE',  ( 13.49999999999999645, 195.4625000012290172, -23.38268590217984766 ) ) ;
#36047=CARTESIAN_POINT ( 'NONE',  ( 27.24356964375000700, 198.1906250006145740, 15.72908226750537075 ) ) ;
#36062=VERTEX_POINT ( 'NONE', #11683 ) ;
#36085=CARTESIAN_POINT ( 'NONE',  ( 5.778771075727756162E-15, 196.7656250006145342, 31.45816453501076637 ) ) ;
#36102=CARTESIAN_POINT ( 'NONE',  ( 27.00000000000000355, 198.4250000000000114, -3.306546357697854128E-15 ) ) ;
#36105=VERTEX_POINT ( 'NONE', #13982 ) ;
#36110=CARTESIAN_POINT ( 'NONE',  ( -26.99999999999999645, 196.4375000000000284, 15.58845726811991561 ) ) ;
#36113=EDGE_CURVE ( 'NONE', #17469, #10453, #30534, .T. ) ;
#36119=CARTESIAN_POINT ( 'NONE',  ( 0.000000000000000000, 200.0000000000000000, 0.000000000000000000 ) ) ;
#36162=CARTESIAN_POINT ( 'NONE',  ( -13.50000000000000533, 195.0875000012290457, -23.38268590217984411 ) ) ;
#36165=( BOUNDED_CURVE ( )  B_SPLINE_CURVE ( 2, ( #12523, #15178, #24086, #23521, #20877, #18220, #26725, #1136, #35631 ),
 .UNSPECIFIED., .F., .F. ) 
 B_SPLINE_CURVE_WITH_KNOTS ( ( 3, 2, 2, 2, 3 ),
 ( 0.1875000000000000000, 0.1944444444444444475, 0.2083333333333333426, 0.2222222222222222099, 0.2291666666666666574 ),
 .UNSPECIFIED. ) 
 CURVE ( )  GEOMETRIC_REPRESENTATION_ITEM ( )  RATIONAL_B_SPLINE_CURVE ( ( 0.9330127018922194093, 0.9330127018922194093, 1.000000000000000000, 0.8660254037844387076, 1.000000000000000000, 0.8660254037844387076, 1.000000000000000000, 0.9330127018922194093, 0.9330127018922194093 ) ) 
 REPRESENTATION_ITEM ( '' )  );
#36192=CARTESIAN_POINT ( 'NONE',  ( -27.24356964375000345, 196.2218750006145456, -15.72908226750537786 ) ) ;
#36204=CARTESIAN_POINT ( 'NONE',  ( 5.778771075727756162E-15, 196.7656250006145342, 31.45816453501075927 ) ) ;
#36217=CARTESIAN_POINT ( 'NONE',  ( -13.50000000000000533, 195.0875000012290457, -23.38268590217984411 ) ) ;
#36232=CARTESIAN_POINT ( 'NONE',  ( 27.24356964374999635, 195.1156250006145001, -15.72908226750539029 ) ) ;
#36245=ORIENTED_EDGE ( 'NONE', *, *, #9709, .T. ) ;
#36257=CARTESIAN_POINT ( 'NONE',  ( -7.234628195640302017, 196.9424038105676971, 27.00000000000000711 ) ) ;
#36267=CARTESIAN_POINT ( 'NONE',  ( 27.24356964374999279, 197.8156250006145171, -15.72908226750539207 ) ) ;
#36283=CARTESIAN_POINT ( 'NONE',  ( -13.49999999999998401, 197.8249999999999886, 23.38268590217985476 ) ) ;
#36298=( NAMED_UNIT ( * ) PLANE_ANGLE_UNIT ( ) SI_UNIT ( $, .RADIAN. ) );
#36303=EDGE_CURVE ( 'NONE', #37392, #33961, #18833, .T. ) ;
#36375=DIRECTION ( 'NONE',  ( 0.000000000000000000, 0.000000000000000000, 1.000000000000000000 ) ) ;
#36379=CARTESIAN_POINT ( 'NONE',  ( 5.778771075727756162E-15, 195.0218750006145569, 31.45816453501076637 ) ) ;
#36387=FACE_OUTER_BOUND ( 'NONE', #31496, .T. ) ;
#36391=CARTESIAN_POINT ( 'NONE',  ( -1.909035429704832693E-15, 199.5500000012290513, -31.17691453623979214 ) ) ;
#36414=CARTESIAN_POINT ( 'NONE',  ( 27.24356964374999635, 196.0156250006145626, -15.72908226750539029 ) ) ;
#36421=VERTEX_POINT ( 'NONE', #29676 ) ;
#36429=VERTEX_POINT ( 'NONE', #29866 ) ;
#36449=ADVANCED_FACE ( 'NONE', ( #3900 ), #35733, .T. ) ;
#36455=CARTESIAN_POINT ( 'NONE',  ( 5.778771075727756162E-15, 197.7218750006145456, 31.45816453501075927 ) ) ;
#36463=ORIENTED_EDGE ( 'NONE', *, *, #12493, .T. ) ;
#36470=CARTESIAN_POINT ( 'NONE',  ( 13.50000000000001421, 197.0000000000000000, 23.38268590217984055 ) ) ;
#36478=CARTESIAN_POINT ( 'NONE',  ( -13.50000000000000533, 199.1375000012290286, -23.38268590217984411 ) ) ;
#36517=VERTEX_POINT ( 'NONE', #10521 ) ;
#36536=EDGE_CURVE ( 'NONE', #4926, #1851, #19268, .T. ) ;
#36547=EDGE_CURVE ( 'NONE', #5600, #1101, #27782, .T. ) ;
#36550=CARTESIAN_POINT ( 'NONE',  ( 1.120210788295102201E-13, 195.5000000012290400, -27.00000000000000711 ) ) ;
#36555=CARTESIAN_POINT ( 'NONE',  ( 0.000000000000000000, 200.0000000000000000, 0.000000000000000000 ) ) ;
#36566=CARTESIAN_POINT ( 'NONE',  ( -13.62178482187498396, 195.8843750006145399, 23.59362340125808188 ) ) ;
#36580=CARTESIAN_POINT ( 'NONE',  ( -13.49999999999998401, 198.8375000012290457, 23.38268590217985476 ) ) ;
#36595=CARTESIAN_POINT ( 'NONE',  ( 0.000000000000000000, 200.0000000000000000, 0.000000000000000000 ) ) ;
#36602=CARTESIAN_POINT ( 'NONE',  ( 5.778771075727756162E-15, 195.4156250006145399, 31.45816453501075927 ) ) ;
#36645=CARTESIAN_POINT ( 'NONE',  ( 27.24356964375000700, 197.7968750006145342, 15.72908226750537075 ) ) ;
#36646=FACE_OUTER_BOUND ( 'NONE', #16582, .T. ) ;
#36656=( NAMED_UNIT ( * ) PLANE_ANGLE_UNIT ( ) SI_UNIT ( $, .RADIAN. ) );
#36662=CARTESIAN_POINT ( 'NONE',  ( 5.727106289114498080E-15, 198.3125000000000000, 31.17691453623979214 ) ) ;
#36663=ORIENTED_EDGE ( 'NONE', *, *, #19096, .F. ) ;
#36688=CARTESIAN_POINT ( 'NONE',  ( -13.50000000000000533, 195.9875000012290229, -23.38268590217984411 ) ) ;
#36751=CARTESIAN_POINT ( 'NONE',  ( 1.069080835302379631E-14, 199.3250000012290286, 27.00000000000000000 ) ) ;
#36757=CARTESIAN_POINT ( 'NONE',  ( -1.926257025242585782E-15, 195.2468750006145513, -31.45816453501076637 ) ) ;
#36767=CARTESIAN_POINT ( 'NONE',  ( -1.909035429704832693E-15, 198.6500000012290457, -31.17691453623979214 ) ) ;
#36780=CARTESIAN_POINT ( 'NONE',  ( 7.234628195640322446, 199.2325961894323711, 26.99999999999999645 ) ) ;
#36788=CARTESIAN_POINT ( 'NONE',  ( 27.24356964375000345, 196.8781250006145171, -3.336375036156643733E-15 ) ) ;
#36829=CARTESIAN_POINT ( 'NONE',  ( -1.926257025242585782E-15, 196.0906250006145228, -31.45816453501076637 ) ) ;
#36830=CARTESIAN_POINT ( 'NONE',  ( -13.62178482187500528, 199.3343750006145569, -23.59362340125807123 ) ) ;
#36832=DIRECTION ( 'NONE',  ( 0.000000000000000000, -0.000000000000000000, -1.000000000000000000 ) ) ;
#36845=CARTESIAN_POINT ( 'NONE',  ( -27.00000000000000355, 196.3625000000000114, -15.58845726811989429 ) ) ;
#36851=CARTESIAN_POINT ( 'NONE',  ( 0.000000000000000000, 200.0000000000000000, 0.000000000000000000 ) ) ;
#36912=CARTESIAN_POINT ( 'NONE',  ( 0.000000000000000000, 200.0000000000000000, 0.000000000000000000 ) ) ;
#36918=CARTESIAN_POINT ( 'NONE',  ( -1.045839947578415010E-13, 195.7250000012290343, 27.00000000000000355 ) ) ;
#36948=CARTESIAN_POINT ( 'NONE',  ( -13.50000000000000533, 197.7875000012290627, -23.38268590217984411 ) ) ;
#36971=VERTEX_POINT ( 'NONE', #18230 ) ;
#36975=EDGE_CURVE ( 'NONE', #32162, #3136, #23911, .T. ) ;
#36976=CARTESIAN_POINT ( 'NONE',  ( 13.62178482187501416, 196.3531250006145115, 23.59362340125806767 ) ) ;
#37001=DIRECTION ( 'NONE',  ( 0.000000000000000000, 0.000000000000000000, -1.000000000000000000 ) ) ;
#37015=CARTESIAN_POINT ( 'NONE',  ( 27.24356964375000700, 198.6968750006145115, 15.72908226750537075 ) ) ;
#37028=CARTESIAN_POINT ( 'NONE',  ( 0.000000000000000000, 2.000000000000000000, 0.000000000000000000 ) ) ;
#37029=CARTESIAN_POINT ( 'NONE',  ( 13.49999999999999645, 195.3500000000000227, -23.38268590217984766 ) ) ;
#37030=ORIENTED_EDGE ( 'NONE', *, *, #32089, .T. ) ;
#37043=EDGE_CURVE ( 'NONE', #32692, #32805, #31646, .T. ) ;
#37069=CARTESIAN_POINT ( 'NONE',  ( 27.00000000000001421, 197.6000000012290627, 15.58845726811988897 ) ) ;
#37073=ORIENTED_EDGE ( 'NONE', *, *, #2314, .F. ) ;
#37107=LINE ( 'NONE', #31246, #37409 ) ;
#37109=DIRECTION ( 'NONE',  ( -0.000000000000000000, -1.000000000000000000, -0.000000000000000000 ) ) ;
#37126=VERTEX_POINT ( 'NONE', #29704 ) ;
#37135=CARTESIAN_POINT ( 'NONE',  ( -26.99999999999998934, 198.8000000012290513, 15.58845726811991561 ) ) ;
#37156=CARTESIAN_POINT ( 'NONE',  ( 1.120210788295102201E-13, 195.3875000000000455, -27.00000000000000711 ) ) ;
#37163=VECTOR ( 'NONE', #33648, 1000.000000000000000 ) ;
#37176=( BOUNDED_CURVE ( )  B_SPLINE_CURVE ( 2, ( #25935, #14377, #26116, #15123, #9064, #5838, #9437, #14564, #34831 ),
 .UNSPECIFIED., .F., .F. ) 
 B_SPLINE_CURVE_WITH_KNOTS ( ( 3, 2, 2, 2, 3 ),
 ( 0.1875000000000000000, 0.1944444444444444475, 0.2083333333333333426, 0.2222222222222222099, 0.2291666666666666574 ),
 .UNSPECIFIED. ) 
 CURVE ( )  GEOMETRIC_REPRESENTATION_ITEM ( )  RATIONAL_B_SPLINE_CURVE ( ( 0.9330127018922194093, 0.9330127018922194093, 1.000000000000000000, 0.8660254037844387076, 1.000000000000000000, 0.8660254037844387076, 1.000000000000000000, 0.9330127018922194093, 0.9330127018922194093 ) ) 
 REPRESENTATION_ITEM ( '' )  );
#37198=CARTESIAN_POINT ( 'NONE',  ( 13.62178482187501416, 195.4531250006145342, 23.59362340125806767 ) ) ;
#37199=CARTESIAN_POINT ( 'NONE',  ( -13.62178482187500528, 197.5343750006145456, -23.59362340125807123 ) ) ;
#37201=CYLINDRICAL_SURFACE ( 'NONE', #16536, 27.00000000000000355 ) ;
#37210=ORIENTED_EDGE ( 'NONE', *, *, #26862, .F. ) ;
#37216=DIRECTION ( 'NONE',  ( 0.000000000000000000, -1.000000000000000000, 0.000000000000000000 ) ) ;
#37217=CARTESIAN_POINT ( 'NONE',  ( 27.00000000000001066, 195.6875000000000000, 15.58845726811988897 ) ) ;
#37250=CARTESIAN_POINT ( 'NONE',  ( 3.253724281355069334E-15, 199.8875000000000455, -27.00000000000000355 ) ) ;
#37255=CARTESIAN_POINT ( 'NONE',  ( 7.234628195640337545, 197.7299038117967029, -26.99999999999999289 ) ) ;
#37297=CARTESIAN_POINT ( 'NONE',  ( -4.694659320240884604E-14, 197.4124999999999943, 27.00000000000000000 ) ) ;
#37318=CARTESIAN_POINT ( 'NONE',  ( 27.00000000000001066, 196.2500000012290116, 15.58845726811988897 ) ) ;
#37331=DIRECTION ( 'NONE',  ( 0.000000000000000000, 0.000000000000000000, -1.000000000000000000 ) ) ;
#37359=CARTESIAN_POINT ( 'NONE',  ( 3.061616997868383043E-15, 2.000000000000000000, 25.00000000000000000 ) ) ;
#37367=CARTESIAN_POINT ( 'NONE',  ( -13.50000000000000533, 196.7750000000000057, -23.38268590217984411 ) ) ;
#37377=CARTESIAN_POINT ( 'NONE',  ( 27.24356964375000700, 195.9968750006145513, 15.72908226750537075 ) ) ;
#37389=CARTESIAN_POINT ( 'NONE',  ( -13.49999999999998401, 196.0250000000000057, 23.38268590217985476 ) ) ;
#37392=VERTEX_POINT ( 'NONE', #17602 ) ;
#37398=CARTESIAN_POINT ( 'NONE',  ( 27.00000000000000355, 195.7250000000000227, -3.306546357697854128E-15 ) ) ;
#37409=VECTOR ( 'NONE', #17224, 1000.000000000000000 ) ;
#37439=ORIENTED_EDGE ( 'NONE', *, *, #5707, .F. ) ;
#37460=CARTESIAN_POINT ( 'NONE',  ( -4.694659320240884604E-14, 197.0750000012290570, 27.00000000000000000 ) ) ;
#37473=CARTESIAN_POINT ( 'NONE',  ( 1.120210788295102201E-13, 196.8500000012290343, -27.00000000000000711 ) ) ;
#37497=CARTESIAN_POINT ( 'NONE',  ( -27.00000000000000355, 196.0250000012290457, -15.58845726811989429 ) ) ;
#37550=COLOUR_RGB('Off White',0.89,0.88,0.83);
#37551=FILL_AREA_STYLE_COLOUR('',#37550);
#37552=FILL_AREA_STYLE('',(#37551));
#37553=SURFACE_STYLE_FILL_AREA(#37552);
#37554=SURFACE_SIDE_STYLE('',(#37553));
#37555=SURFACE_STYLE_USAGE(.BOTH.,#37554);
#37556=PRESENTATION_STYLE_ASSIGNMENT((#37555));
ENDSEC;
END-ISO-10303-21;
